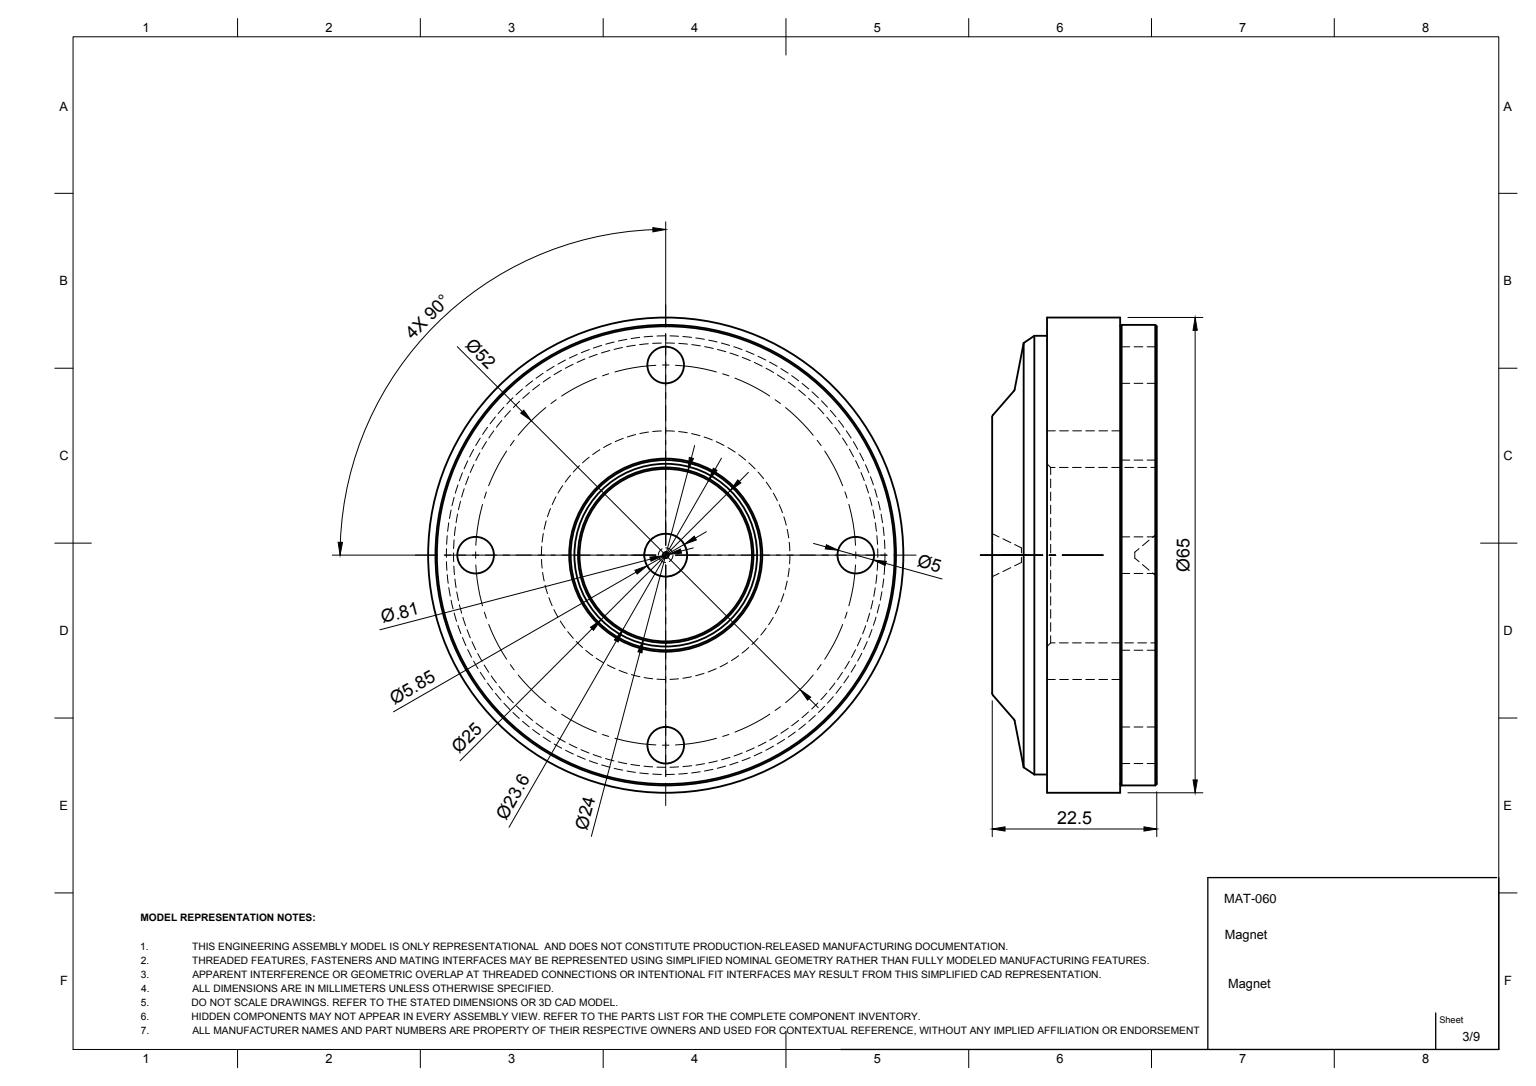
ISO-10303-21;
HEADER;
FILE_DESCRIPTION (('STEP AP214'),
    '1' );
FILE_NAME ('Magnet.step',
    '2026-10-29T23:46:56',
    ( '' ),
    ( '' ),
    'SwSTEP 2.0',
    'SolidWorks 2020',
    '' );
FILE_SCHEMA (( 'AUTOMOTIVE_DESIGN' ));
ENDSEC;

DATA;
#2=VECTOR ( 'NONE', #10897, 1000.000000000000000 ) ;
#14=CONICAL_SURFACE ( 'NONE', #3681, 2.923537884824412014, 0.6981317007977324574 ) ;
#45=AXIS2_PLACEMENT_3D ( 'NONE', #7239, #26769, #16743 ) ;
#47=VECTOR ( 'NONE', #22684, 1000.000000000000114 ) ;
#71=ORIENTED_EDGE ( 'NONE', *, *, #26696, .T. ) ;
#91=AXIS2_PLACEMENT_3D ( 'NONE', #3983, #26796, #16125 ) ;
#98=CONICAL_SURFACE ( 'NONE', #18421, 11.79999999999997762, 0.7853981633974786991 ) ;
#100=VECTOR ( 'NONE', #2675, 1000.000000000000114 ) ;
#109=FACE_OUTER_BOUND ( 'NONE', #5838, .T. ) ;
#111=DIRECTION ( 'NONE',  ( -0.000000000000000000, 1.000000000000000000, -0.000000000000000000 ) ) ;
#122=EDGE_CURVE ( 'NONE', #19617, #28878, #29198, .T. ) ;
#132=DIRECTION ( 'NONE',  ( 0.000000000000000000, 0.000000000000000000, -1.000000000000000000 ) ) ;
#244=VECTOR ( 'NONE', #7734, 1000.000000000000114 ) ;
#252=LINE ( 'NONE', #27506, #6964 ) ;
#257=VERTEX_POINT ( 'NONE', #4514 ) ;
#265=FACE_OUTER_BOUND ( 'NONE', #5953, .T. ) ;
#277=ORIENTED_EDGE ( 'NONE', *, *, #29434, .F. ) ;
#296=AXIS2_PLACEMENT_3D ( 'NONE', #20204, #23316, #10529 ) ;
#298=EDGE_CURVE ( 'NONE', #8568, #25382, #4926, .T. ) ;
#348=DIRECTION ( 'NONE',  ( -0.000000000000000000, -1.000000000000000000, -0.000000000000000000 ) ) ;
#447=ORIENTED_EDGE ( 'NONE', *, *, #29161, .T. ) ;
#459=ORIENTED_EDGE ( 'NONE', *, *, #23712, .T. ) ;
#483=ADVANCED_FACE ( 'NONE', ( #7004 ), #4048, .T. ) ;
#496=LINE ( 'NONE', #32361, #244 ) ;
#502=DIRECTION ( 'NONE',  ( 0.000000000000000000, 0.000000000000000000, 1.000000000000000000 ) ) ;
#538=ORIENTED_EDGE ( 'NONE', *, *, #31344, .T. ) ;
#605=DIRECTION ( 'NONE',  ( 0.000000000000000000, -1.000000000000000000, 0.000000000000000000 ) ) ;
#622=CIRCLE ( 'NONE', #1640, 30.00000000000000000 ) ;
#636=FACE_OUTER_BOUND ( 'NONE', #28736, .T. ) ;
#638=ORIENTED_EDGE ( 'NONE', *, *, #25897, .T. ) ;
#686=ORIENTED_EDGE ( 'NONE', *, *, #11571, .F. ) ;
#691=ORIENTED_EDGE ( 'NONE', *, *, #20114, .F. ) ;
#732=ORIENTED_EDGE ( 'NONE', *, *, #12775, .F. ) ;
#759=PLANE ( 'NONE',  #9679 ) ;
#765=CARTESIAN_POINT ( 'NONE',  ( 21.09785597605719332, 30.56454579224779522, 47.04930799450051637 ) ) ;
#768=DIRECTION ( 'NONE',  ( -0.000000000000000000, -1.000000000000000000, -0.000000000000000000 ) ) ;
#814=CYLINDRICAL_SURFACE ( 'NONE', #19867, 2.499999999999998668 ) ;
#816=EDGE_LOOP ( 'NONE', ( #11067, #9782, #2400, #22463 ) ) ;
#819=ADVANCED_FACE ( 'NONE', ( #7090 ), #4794, .F. ) ;
#883=CARTESIAN_POINT ( 'NONE',  ( 21.09785597605719332, 30.56454579224779522, 47.04930799450051637 ) ) ;
#932=ORIENTED_EDGE ( 'NONE', *, *, #25282, .F. ) ;
#939=AXIS2_PLACEMENT_3D ( 'NONE', #4537, #12591, #24892 ) ;
#952=VECTOR ( 'NONE', #28444, 1000.000000000000114 ) ;
#1011=CARTESIAN_POINT ( 'NONE',  ( 21.09785597605719687, 43.75535478762431296, 76.06768081105269630 ) ) ;
#1060=ORIENTED_EDGE ( 'NONE', *, *, #12224, .F. ) ;
#1066=STYLED_ITEM('',(#32522),#12454);
#1071=ORIENTED_EDGE ( 'NONE', *, *, #23936, .F. ) ;
#1082=CARTESIAN_POINT ( 'NONE',  ( 21.09785597605719332, 40.56454579224780588, 47.04930799450051637 ) ) ;
#1089=EDGE_LOOP ( 'NONE', ( #31480, #28380, #1599, #4895 ) ) ;
#1092=CARTESIAN_POINT ( 'NONE',  ( 21.09785597605719332, 40.06454579224778456, 47.04930799450051637 ) ) ;
#1118=EDGE_LOOP ( 'NONE', ( #1286, #26031, #11888, #26251 ) ) ;
#1132=AXIS2_PLACEMENT_3D ( 'NONE', #16655, #9285, #24220 ) ;
#1146=CIRCLE ( 'NONE', #29981, 12.50000000000001776 ) ;
#1173=VECTOR ( 'NONE', #9327, 1000.000000000000000 ) ;
#1185=ADVANCED_FACE ( 'NONE', ( #16721 ), #7215, .T. ) ;
#1203=EDGE_LOOP ( 'NONE', ( #5817, #15284, #10647, #19677 ) ) ;
#1217=VECTOR ( 'NONE', #18449, 1000.000000000000000 ) ;
#1226=CARTESIAN_POINT ( 'NONE',  ( 21.09785597605719332, 30.36454579224779238, 47.04930799450051637 ) ) ;
#1235=DIRECTION ( 'NONE',  ( 0.000000000000000000, 0.000000000000000000, 1.000000000000000000 ) ) ;
#1286=ORIENTED_EDGE ( 'NONE', *, *, #27316, .F. ) ;
#1292=EDGE_LOOP ( 'NONE', ( #17485, #2942, #9544, #30462 ) ) ;
#1300=AXIS2_PLACEMENT_3D ( 'NONE', #24449, #4434, #31842 ) ;
#1313=EDGE_LOOP ( 'NONE', ( #3808, #4252, #18593, #32168 ) ) ;
#1333=COLOUR_RGB ( '',0.7921568627450980005, 0.8196078431372548767, 0.9333333333333333481 ) ;
#1342=CARTESIAN_POINT ( 'NONE',  ( 21.09785597605719332, 30.56454579224779522, 15.74930799450053520 ) ) ;
#1354=DIRECTION ( 'NONE',  ( 0.000000000000000000, 0.000000000000000000, 1.000000000000000000 ) ) ;
#1359=EDGE_CURVE ( 'NONE', #12063, #12175, #10176, .T. ) ;
#1389=CARTESIAN_POINT ( 'NONE',  ( 21.09785597605719332, 30.56454579224779522, 33.84930799450050642 ) ) ;
#1408=DIRECTION ( 'NONE',  ( -0.000000000000000000, 1.000000000000000000, -0.000000000000000000 ) ) ;
#1416=EDGE_CURVE ( 'NONE', #25267, #14096, #7468, .T. ) ;
#1442=DIRECTION ( 'NONE',  ( 0.000000000000000000, 0.000000000000000000, 1.000000000000000000 ) ) ;
#1444=AXIS2_PLACEMENT_3D ( 'NONE', #20383, #7445, #27619 ) ;
#1449=EDGE_LOOP ( 'NONE', ( #4769, #28960 ) ) ;
#1462=DIRECTION ( 'NONE',  ( 0.000000000000000000, 0.000000000000000000, -1.000000000000000000 ) ) ;
#1504=DIRECTION ( 'NONE',  ( 0.000000000000000000, -0.000000000000000000, -1.000000000000000000 ) ) ;
#1516=FILL_AREA_STYLE ('',( #3660 ) ) ;
#1564=VERTEX_POINT ( 'NONE', #24406 ) ;
#1575=ORIENTED_EDGE ( 'NONE', *, *, #22675, .F. ) ;
#1598=AXIS2_PLACEMENT_3D ( 'NONE', #20368, #5295, #15139 ) ;
#1599=ORIENTED_EDGE ( 'NONE', *, *, #28935, .T. ) ;
#1601=PLANE ( 'NONE',  #30450 ) ;
#1625=AXIS2_PLACEMENT_3D ( 'NONE', #26803, #31574, #31889 ) ;
#1633=ORIENTED_EDGE ( 'NONE', *, *, #8614, .T. ) ;
#1640=AXIS2_PLACEMENT_3D ( 'NONE', #1082, #605, #20783 ) ;
#1645=AXIS2_PLACEMENT_3D ( 'NONE', #2215, #7303, #27489 ) ;
#1727=DIRECTION ( 'NONE',  ( 0.000000000000000000, 0.000000000000000000, 1.000000000000000000 ) ) ;
#1779=EDGE_CURVE ( 'NONE', #24681, #28894, #7495, .T. ) ;
#1787=DIRECTION ( 'NONE',  ( 0.000000000000000000, 0.000000000000000000, -1.000000000000000000 ) ) ;
#1790=VERTEX_POINT ( 'NONE', #20937 ) ;
#1801=EDGE_CURVE ( 'NONE', #17244, #15830, #19463, .T. ) ;
#1816=EDGE_CURVE ( 'NONE', #22757, #5318, #622, .T. ) ;
#1839=ADVANCED_FACE ( 'NONE', ( #31129, #10942 ), #30649, .T. ) ;
#1877=AXIS2_PLACEMENT_3D ( 'NONE', #16713, #9184, #26743 ) ;
#1887=FACE_OUTER_BOUND ( 'NONE', #17720, .T. ) ;
#1919=EDGE_LOOP ( 'NONE', ( #1575, #9249, #30657, #15820 ) ) ;
#1961=AXIS2_PLACEMENT_3D ( 'NONE', #13939, #11633, #11953 ) ;
#1975=ORIENTED_EDGE ( 'NONE', *, *, #7569, .F. ) ;
#1985=EDGE_CURVE ( 'NONE', #6454, #6391, #27880, .T. ) ;
#1987=AXIS2_PLACEMENT_3D ( 'NONE', #8912, #6617, #21212 ) ;
#2008=FACE_OUTER_BOUND ( 'NONE', #5670, .T. ) ;
#2035=EDGE_LOOP ( 'NONE', ( #28490, #17099, #19281, #32413 ) ) ;
#2068=AXIS2_PLACEMENT_3D ( 'NONE', #7531, #10318, #15399 ) ;
#2095=DIRECTION ( 'NONE',  ( 0.000000000000000000, 0.000000000000000000, -1.000000000000000000 ) ) ;
#2121=DIRECTION ( 'NONE',  ( -0.000000000000000000, -1.000000000000000000, -0.000000000000000000 ) ) ;
#2136=DIRECTION ( 'NONE',  ( 0.000000000000000000, 1.000000000000000000, 0.000000000000000000 ) ) ;
#2162=DIRECTION ( 'NONE',  ( 0.000000000000000000, 0.000000000000000000, 1.000000000000000000 ) ) ;
#2215=CARTESIAN_POINT ( 'NONE',  ( 21.09785597605719332, 30.36454579224779238, 47.04930799450051637 ) ) ;
#2245=FACE_BOUND ( 'NONE', #17285, .T. ) ;
#2286=VERTEX_POINT ( 'NONE', #12813 ) ;
#2314=PLANE ( 'NONE',  #32485 ) ;
#2325=AXIS2_PLACEMENT_3D ( 'NONE', #7259, #22180, #32208 ) ;
#2337=DIRECTION ( 'NONE',  ( 0.000000000000000000, 1.000000000000000000, 0.000000000000000000 ) ) ;
#2354=ORIENTED_EDGE ( 'NONE', *, *, #13031, .T. ) ;
#2355=EDGE_LOOP ( 'NONE', ( #9054, #15659, #16923, #25728 ) ) ;
#2360=AXIS2_PLACEMENT_3D ( 'NONE', #29508, #9641, #14246 ) ;
#2389=CARTESIAN_POINT ( 'NONE',  ( 21.09785597605719332, 25.56454579224779167, 33.84930799450050642 ) ) ;
#2400=ORIENTED_EDGE ( 'NONE', *, *, #2953, .T. ) ;
#2406=CARTESIAN_POINT ( 'NONE',  ( 21.09785597605719332, 48.06454579224779877, 50.00023834876391504 ) ) ;
#2432=EDGE_CURVE ( 'NONE', #5318, #19617, #8358, .T. ) ;
#2438=ORIENTED_EDGE ( 'NONE', *, *, #7569, .T. ) ;
#2466=EDGE_LOOP ( 'NONE', ( #32496, #15726, #538, #3563 ) ) ;
#2498=CARTESIAN_POINT ( 'NONE',  ( 21.09785597605719332, 40.06454579224778456, 59.04930799450051637 ) ) ;
#2505=ORIENTED_EDGE ( 'NONE', *, *, #17038, .T. ) ;
#2580=DIRECTION ( 'NONE',  ( 0.000000000000000000, 0.000000000000000000, -1.000000000000000000 ) ) ;
#2598=EDGE_CURVE ( 'NONE', #23536, #19811, #3820, .T. ) ;
#2626=ORIENTED_EDGE ( 'NONE', *, *, #122, .T. ) ;
#2658=FACE_OUTER_BOUND ( 'NONE', #25338, .T. ) ;
#2674=FACE_OUTER_BOUND ( 'NONE', #2355, .T. ) ;
#2675=DIRECTION ( 'NONE',  ( 9.242526717056601033E-17, -0.6560590289905074979, 0.7547095802227717920 ) ) ;
#2699=LINE ( 'NONE', #15019, #27764 ) ;
#2784=FACE_OUTER_BOUND ( 'NONE', #1292, .T. ) ;
#2814=EDGE_CURVE ( 'NONE', #4198, #16034, #19041, .T. ) ;
#2856=AXIS2_PLACEMENT_3D ( 'NONE', #24398, #17003, #21928 ) ;
#2867=ORIENTED_EDGE ( 'NONE', *, *, #8743, .T. ) ;
#2878=PRODUCT_DEFINITION_CONTEXT ( 'detailed design', #25444, 'design' ) ;
#2879=ORIENTED_EDGE ( 'NONE', *, *, #8848, .F. ) ;
#2893=FACE_BOUND ( 'NONE', #21626, .T. ) ;
#2924=EDGE_CURVE ( 'NONE', #9356, #12175, #6500, .T. ) ;
#2935=CIRCLE ( 'NONE', #15520, 13.00000000000000533 ) ;
#2942=ORIENTED_EDGE ( 'NONE', *, *, #6749, .F. ) ;
#2953=EDGE_CURVE ( 'NONE', #25453, #12063, #26847, .T. ) ;
#3023=CARTESIAN_POINT ( 'NONE',  ( 21.09785597605719687, 40.56454579224780588, 17.04930799450051637 ) ) ;
#3047=CARTESIAN_POINT ( 'NONE',  ( 21.09785597605719332, 42.30003263981368633, 47.04930799450051637 ) ) ;
#3112=CIRCLE ( 'NONE', #23030, 2.950930354263400890 ) ;
#3168=CARTESIAN_POINT ( 'NONE',  ( 21.09785597605719332, 25.56454579224779877, 47.04930799450051637 ) ) ;
#3178=CYLINDRICAL_SURFACE ( 'NONE', #10556, 2.500000000000002220 ) ;
#3199=AXIS2_PLACEMENT_3D ( 'NONE', #4469, #4630, #11701 ) ;
#3200=ADVANCED_FACE ( 'NONE', ( #4853 ), #25367, .F. ) ;
#3211=FACE_OUTER_BOUND ( 'NONE', #19132, .T. ) ;
#3215=ORIENTED_EDGE ( 'NONE', *, *, #6112, .T. ) ;
#3220=CARTESIAN_POINT ( 'NONE',  ( 21.09785597605719332, 30.56454579224779522, 73.04930799450052348 ) ) ;
#3299=PRODUCT ( 'Magnet', 'Magnet', '', ( #30204 ) ) ;
#3304=EDGE_LOOP ( 'NONE', ( #14921, #19098, #10073, #24712 ) ) ;
#3352=ORIENTED_EDGE ( 'NONE', *, *, #29648, .F. ) ;
#3370=ORIENTED_EDGE ( 'NONE', *, *, #21556, .T. ) ;
#3379=DIRECTION ( 'NONE',  ( 0.000000000000000000, -1.000000000000000000, 0.000000000000000000 ) ) ;
#3382=DIRECTION ( 'NONE',  ( -0.000000000000000000, -1.000000000000000000, -0.000000000000000000 ) ) ;
#3393=AXIS2_PLACEMENT_3D ( 'NONE', #22988, #25620, #502 ) ;
#3400=ADVANCED_FACE ( 'NONE', ( #20590 ), #13812, .T. ) ;
#3464=CARTESIAN_POINT ( 'NONE',  ( 21.09785597605719332, 25.56454579224779877, 49.97284587932492883 ) ) ;
#3500=DIRECTION ( 'NONE',  ( 0.000000000000000000, 0.000000000000000000, -1.000000000000000000 ) ) ;
#3529=ORIENTED_EDGE ( 'NONE', *, *, #7650, .F. ) ;
#3532=CARTESIAN_POINT ( 'NONE',  ( 21.09785597605719332, 25.56454579224779877, 47.04930799450051637 ) ) ;
#3563=ORIENTED_EDGE ( 'NONE', *, *, #8136, .T. ) ;
#3615=ORIENTED_EDGE ( 'NONE', *, *, #29434, .T. ) ;
#3660=FILL_AREA_STYLE_COLOUR ( '', #1333 ) ;
#3680=AXIS2_PLACEMENT_3D ( 'NONE', #5413, #15417, #25429 ) ;
#3681=AXIS2_PLACEMENT_3D ( 'NONE', #15156, #32392, #29939 ) ;
#3719=VECTOR ( 'NONE', #16013, 1000.000000000000000 ) ;
#3727=TOROIDAL_SURFACE ( 'NONE', #6353, 18.86195243859455672, 0.5000000000000000000 ) ;
#3731=CIRCLE ( 'NONE', #12060, 31.29999999999997229 ) ;
#3738=VERTEX_POINT ( 'NONE', #21023 ) ;
#3745=LINE ( 'NONE', #11304, #27933 ) ;
#3765=ORIENTED_EDGE ( 'NONE', *, *, #1816, .F. ) ;
#3768=FACE_OUTER_BOUND ( 'NONE', #18350, .T. ) ;
#3769=CARTESIAN_POINT ( 'NONE',  ( -4.902144023942810236, 30.56554579224779644, 44.54930799450042400 ) ) ;
#3808=ORIENTED_EDGE ( 'NONE', *, *, #30736, .F. ) ;
#3811=CARTESIAN_POINT ( 'NONE',  ( 21.09785597605719332, 30.36454579224777461, 15.54930799450051460 ) ) ;
#3820=CIRCLE ( 'NONE', #21121, 2.500000000000002220 ) ;
#3823=( NAMED_UNIT ( * ) PLANE_ANGLE_UNIT ( ) SI_UNIT ( $, .RADIAN. ) );
#3844=ADVANCED_FACE ( 'NONE', ( #32351 ), #2314, .T. ) ;
#3848=AXIS2_PLACEMENT_3D ( 'NONE', #29111, #24333, #22031 ) ;
#3870=DIRECTION ( 'NONE',  ( 0.000000000000000000, 1.000000000000000000, 0.000000000000000000 ) ) ;
#3872=DIRECTION ( 'NONE',  ( 8.659560562354931626E-17, 0.7071067811865474617, -0.7071067811865475727 ) ) ;
#3881=ORIENTED_EDGE ( 'NONE', *, *, #14421, .F. ) ;
#3913=CARTESIAN_POINT ( 'NONE',  ( 21.09785597605719332, 44.06454579224779877, 47.04930799450051637 ) ) ;
#3917=AXIS2_PLACEMENT_3D ( 'NONE', #15584, #10691, #25602 ) ;
#3919=CARTESIAN_POINT ( 'NONE',  ( 21.09785597605719332, 30.36454579224779238, 34.04930799450050927 ) ) ;
#3922=DIRECTION ( 'NONE',  ( -0.000000000000000000, -1.000000000000000000, -0.000000000000000000 ) ) ;
#3952=VERTEX_POINT ( 'NONE', #10829 ) ;
#3983=CARTESIAN_POINT ( 'NONE',  ( 21.09785597605719332, 44.06454579224779877, 47.04930799450051637 ) ) ;
#3987=FACE_OUTER_BOUND ( 'NONE', #11241, .T. ) ;
#3988=EDGE_CURVE ( 'NONE', #7332, #10562, #29362, .T. ) ;
#3991=DIRECTION ( 'NONE',  ( 0.000000000000000000, 0.000000000000000000, -1.000000000000000000 ) ) ;
#3998=DIRECTION ( 'NONE',  ( 1.202146588165213953E-16, -0.1908089953765421121, 0.9816271834476645308 ) ) ;
#4013=CARTESIAN_POINT ( 'NONE',  ( 47.09785597605719687, 30.56554579224779644, 49.54930799450078638 ) ) ;
#4043=ORIENTED_EDGE ( 'NONE', *, *, #23890, .F. ) ;
#4048=PLANE ( 'NONE',  #18437 ) ;
#4100=DIRECTION ( 'NONE',  ( 0.000000000000000000, 0.000000000000000000, -1.000000000000000000 ) ) ;
#4115=ORIENTED_EDGE ( 'NONE', *, *, #25644, .T. ) ;
#4149=EDGE_CURVE ( 'NONE', #19482, #30996, #10519, .T. ) ;
#4181=DIRECTION ( 'NONE',  ( 0.000000000000000000, 0.000000000000000000, 1.000000000000000000 ) ) ;
#4185=ORIENTED_EDGE ( 'NONE', *, *, #15938, .T. ) ;
#4198=VERTEX_POINT ( 'NONE', #19641 ) ;
#4211=VECTOR ( 'NONE', #12710, 1000.000000000000000 ) ;
#4219=EDGE_LOOP ( 'NONE', ( #12264, #18361, #29054, #29638 ) ) ;
#4221=ADVANCED_FACE ( 'NONE', ( #22270 ), #14159, .T. ) ;
#4222=DIRECTION ( 'NONE',  ( -0.000000000000000000, -1.000000000000000000, -0.000000000000000000 ) ) ;
#4225=DIRECTION ( 'NONE',  ( -0.000000000000000000, 1.000000000000000000, -0.000000000000000000 ) ) ;
#4251=DIRECTION ( 'NONE',  ( 0.000000000000000000, -1.000000000000000000, 0.000000000000000000 ) ) ;
#4252=ORIENTED_EDGE ( 'NONE', *, *, #2598, .F. ) ;
#4295=DIRECTION ( 'NONE',  ( 0.000000000000000000, 0.000000000000000000, 1.000000000000000000 ) ) ;
#4304=AXIS2_PLACEMENT_3D ( 'NONE', #7479, #29300, #27003 ) ;
#4310=AXIS2_PLACEMENT_3D ( 'NONE', #3532, #16931, #19222 ) ;
#4318=CARTESIAN_POINT ( 'NONE',  ( 21.09785597605719332, 40.56454579224779877, 47.04930799450051637 ) ) ;
#4336=CONICAL_SURFACE ( 'NONE', #15873, 31.29999999999997939, 0.7853981633974482790 ) ;
#4397=DIRECTION ( 'NONE',  ( 0.000000000000000000, 0.000000000000000000, 1.000000000000000000 ) ) ;
#4434=DIRECTION ( 'NONE',  ( 0.000000000000000000, 1.000000000000000000, 0.000000000000000000 ) ) ;
#4454=AXIS2_PLACEMENT_3D ( 'NONE', #22592, #111, #27854 ) ;
#4458=DIRECTION ( 'NONE',  ( 0.000000000000000000, -1.000000000000000000, 0.000000000000000000 ) ) ;
#4459=DIRECTION ( 'NONE',  ( -1.000000000000000000, 0.000000000000000000, 0.000000000000000000 ) ) ;
#4468=CARTESIAN_POINT ( 'NONE',  ( 21.09785597605719332, 47.94190058235918173, 47.04930799450051637 ) ) ;
#4469=CARTESIAN_POINT ( 'NONE',  ( 21.09785597605719332, 30.56454579224779522, 47.04930799450051637 ) ) ;
#4509=DIRECTION ( 'NONE',  ( 0.000000000000000000, 0.000000000000000000, 1.000000000000000000 ) ) ;
#4514=CARTESIAN_POINT ( 'NONE',  ( 21.09785597605719332, 25.56454579224779167, 60.24930799450052632 ) ) ;
#4523=ORIENTED_EDGE ( 'NONE', *, *, #1416, .F. ) ;
#4537=CARTESIAN_POINT ( 'NONE',  ( 21.09785597605719332, 25.56454579224779167, 47.04930799450051637 ) ) ;
#4575=EDGE_CURVE ( 'NONE', #14096, #28333, #31930, .T. ) ;
#4603=DIRECTION ( 'NONE',  ( 0.000000000000000000, -1.000000000000000000, 0.000000000000000000 ) ) ;
#4610=AXIS2_PLACEMENT_3D ( 'NONE', #31469, #23749, #11436 ) ;
#4630=DIRECTION ( 'NONE',  ( 0.000000000000000000, -1.000000000000000000, 0.000000000000000000 ) ) ;
#4650=DIRECTION ( 'NONE',  ( 0.000000000000000000, 0.000000000000000000, -1.000000000000000000 ) ) ;
#4661=AXIS2_PLACEMENT_3D ( 'NONE', #16707, #4251, #5184 ) ;
#4765=DIRECTION ( 'NONE',  ( 0.000000000000000000, 0.000000000000000000, -1.000000000000000000 ) ) ;
#4769=ORIENTED_EDGE ( 'NONE', *, *, #26658, .T. ) ;
#4778=CIRCLE ( 'NONE', #23111, 0.5000000000000004441 ) ;
#4792=CONICAL_SURFACE ( 'NONE', #91, 0.9999999999999731326, 0.4537856055185219284 ) ;
#4794=CYLINDRICAL_SURFACE ( 'NONE', #22047, 16.99999999999999289 ) ;
#4840=LINE ( 'NONE', #27973, #2 ) ;
#4848=PLANE ( 'NONE',  #4304 ) ;
#4853=FACE_OUTER_BOUND ( 'NONE', #31799, .T. ) ;
#4871=ORIENTED_EDGE ( 'NONE', *, *, #3988, .F. ) ;
#4893=CARTESIAN_POINT ( 'NONE',  ( 21.09785597605719687, 45.28940914544685370, 24.35070776595075515 ) ) ;
#4895=ORIENTED_EDGE ( 'NONE', *, *, #27999, .T. ) ;
#4914=ORIENTED_EDGE ( 'NONE', *, *, #28935, .F. ) ;
#4926=CIRCLE ( 'NONE', #20118, 31.50000000000000711 ) ;
#4931=ORIENTED_EDGE ( 'NONE', *, *, #31027, .T. ) ;
#4962=DIRECTION ( 'NONE',  ( -0.000000000000000000, -1.000000000000000000, -0.000000000000000000 ) ) ;
#5016=CARTESIAN_POINT ( 'NONE',  ( 21.09785597605719332, 25.76454579224776964, 47.04930799450051637 ) ) ;
#5060=CARTESIAN_POINT ( 'NONE',  ( 21.09785597605719332, 40.56454579224780588, 77.04930799450052348 ) ) ;
#5081=DIRECTION ( 'NONE',  ( -0.000000000000000000, 1.000000000000000000, 0.000000000000000000 ) ) ;
#5129=CYLINDRICAL_SURFACE ( 'NONE', #1598, 16.99999999999999289 ) ;
#5175=AXIS2_PLACEMENT_3D ( 'NONE', #26946, #23831, #1504 ) ;
#5178=CARTESIAN_POINT ( 'NONE',  ( 21.09785597605719332, 43.75535478762431296, 47.04930799450051637 ) ) ;
#5184=DIRECTION ( 'NONE',  ( 0.000000000000000000, 0.000000000000000000, -1.000000000000000000 ) ) ;
#5193=CARTESIAN_POINT ( 'NONE',  ( 21.09785597605719332, 25.56454579224779167, 60.24930799450052632 ) ) ;
#5195=VERTEX_POINT ( 'NONE', #21791 ) ;
#5208=VERTEX_POINT ( 'NONE', #19324 ) ;
#5209=FACE_OUTER_BOUND ( 'NONE', #14516, .T. ) ;
#5272=CIRCLE ( 'NONE', #28838, 2.500000000000002220 ) ;
#5295=DIRECTION ( 'NONE',  ( -0.000000000000000000, 1.000000000000000000, -0.000000000000000000 ) ) ;
#5318=VERTEX_POINT ( 'NONE', #5060 ) ;
#5338=DIRECTION ( 'NONE',  ( 0.000000000000000000, -1.000000000000000000, 0.000000000000000000 ) ) ;
#5413=CARTESIAN_POINT ( 'NONE',  ( 21.09785597605719332, 25.56454579224779167, 21.04930799450051282 ) ) ;
#5435=ORIENTED_EDGE ( 'NONE', *, *, #12257, .F. ) ;
#5489=VECTOR ( 'NONE', #32288, 1000.000000000000114 ) ;
#5554=VERTEX_POINT ( 'NONE', #10802 ) ;
#5606=CARTESIAN_POINT ( 'NONE',  ( 21.09785597605719332, 25.56454579224779877, 47.04930799450051637 ) ) ;
#5654=DIRECTION ( 'NONE',  ( -0.000000000000000000, -1.000000000000000000, -0.000000000000000000 ) ) ;
#5661=FACE_OUTER_BOUND ( 'NONE', #23654, .T. ) ;
#5670=EDGE_LOOP ( 'NONE', ( #9048, #26323, #27618, #15172 ) ) ;
#5672=AXIS2_PLACEMENT_3D ( 'NONE', #9629, #22745, #29655 ) ;
#5688=DIRECTION ( 'NONE',  ( 0.000000000000000000, -1.000000000000000000, 0.000000000000000000 ) ) ;
#5736=CARTESIAN_POINT ( 'NONE',  ( 21.09785597605719332, 44.99492099041257376, 47.04930799450051637 ) ) ;
#5741=CARTESIAN_POINT ( 'NONE',  ( 21.09785597605719332, 43.75535478762431296, 47.04930799450051637 ) ) ;
#5748=VECTOR ( 'NONE', #3998, 1000.000000000000000 ) ;
#5789=CARTESIAN_POINT ( 'NONE',  ( 21.09785597605719687, 30.56454579224779522, 14.54930799450051460 ) ) ;
#5811=AXIS2_PLACEMENT_3D ( 'NONE', #21100, #11116, #13265 ) ;
#5817=ORIENTED_EDGE ( 'NONE', *, *, #6229, .F. ) ;
#5838=EDGE_LOOP ( 'NONE', ( #12861, #28090, #20021, #25579 ) ) ;
#5855=AXIS2_PLACEMENT_3D ( 'NONE', #23260, #10799, #15876 ) ;
#5874=DIRECTION ( 'NONE',  ( -0.000000000000000000, -1.000000000000000000, -0.000000000000000000 ) ) ;
#5907=DIRECTION ( 'NONE',  ( 0.000000000000000000, 0.000000000000000000, -1.000000000000000000 ) ) ;
#5935=CONICAL_SURFACE ( 'NONE', #32123, 12.00000000000000355, 0.7853981633974466137 ) ;
#5953=EDGE_LOOP ( 'NONE', ( #24646, #2867, #26798, #22358 ) ) ;
#5977=DIRECTION ( 'NONE',  ( 1.000000000000000000, 0.000000000000000000, 0.000000000000000000 ) ) ;
#5997=AXIS2_PLACEMENT_3D ( 'NONE', #21521, #8734, #18731 ) ;
#6017=DIRECTION ( 'NONE',  ( 0.000000000000000000, -0.000000000000000000, 1.000000000000000000 ) ) ;
#6032=CIRCLE ( 'NONE', #3393, 2.950930354263400890 ) ;
#6034=CARTESIAN_POINT ( 'NONE',  ( 21.09785597605719332, 25.56454579224779167, 33.84930799450050642 ) ) ;
#6063=FACE_BOUND ( 'NONE', #12293, .T. ) ;
#6112=EDGE_CURVE ( 'NONE', #19482, #20710, #16307, .T. ) ;
#6113=ORIENTED_EDGE ( 'NONE', *, *, #12775, .T. ) ;
#6130=DIRECTION ( 'NONE',  ( -0.000000000000000000, -1.000000000000000000, -0.000000000000000000 ) ) ;
#6164=EDGE_LOOP ( 'NONE', ( #459, #13899 ) ) ;
#6229=EDGE_CURVE ( 'NONE', #15830, #17244, #19880, .T. ) ;
#6286=CARTESIAN_POINT ( 'NONE',  ( 0.000000000000000000, 0.000000000000000000, 0.000000000000000000 ) ) ;
#6310=ORIENTED_EDGE ( 'NONE', *, *, #29829, .T. ) ;
#6311=VECTOR ( 'NONE', #15099, 1000.000000000000227 ) ;
#6322=FACE_OUTER_BOUND ( 'NONE', #14016, .T. ) ;
#6353=AXIS2_PLACEMENT_3D ( 'NONE', #12902, #19938, #25032 ) ;
#6370=AXIS2_PLACEMENT_3D ( 'NONE', #30165, #3382, #23412 ) ;
#6379=EDGE_LOOP ( 'NONE', ( #12720, #25399, #4185, #71 ) ) ;
#6391=VERTEX_POINT ( 'NONE', #25600 ) ;
#6440=ORIENTED_EDGE ( 'NONE', *, *, #22675, .T. ) ;
#6454=VERTEX_POINT ( 'NONE', #15112 ) ;
#6483=DIRECTION ( 'NONE',  ( 0.000000000000000000, 0.000000000000000000, -1.000000000000000000 ) ) ;
#6500=CIRCLE ( 'NONE', #7562, 12.00000000000000355 ) ;
#6510=UNCERTAINTY_MEASURE_WITH_UNIT (LENGTH_MEASURE( 1.000000000000000082E-05 ), #21204, 'distance_accuracy_value', 'NONE');
#6545=CIRCLE ( 'NONE', #4454, 22.50178251985260758 ) ;
#6562=CARTESIAN_POINT ( 'NONE',  ( 21.09785597605719687, 40.56454579224779877, 30.04930799450051282 ) ) ;
#6604=PLANE ( 'NONE',  #5175 ) ;
#6617=DIRECTION ( 'NONE',  ( 0.000000000000000000, 1.000000000000000000, 0.000000000000000000 ) ) ;
#6636=EDGE_CURVE ( 'NONE', #24883, #22063, #9895, .T. ) ;
#6653=AXIS2_PLACEMENT_3D ( 'NONE', #27542, #5654, #132 ) ;
#6710=EDGE_CURVE ( 'NONE', #25964, #25453, #10441, .T. ) ;
#6732=CARTESIAN_POINT ( 'NONE',  ( 21.09785597605719332, 30.56454579224779522, 15.54930799450051460 ) ) ;
#6749=EDGE_CURVE ( 'NONE', #12175, #9356, #27718, .T. ) ;
#6812=DIRECTION ( 'NONE',  ( 1.000000000000000000, 0.000000000000000000, 2.775557561562892534E-15 ) ) ;
#6843=VECTOR ( 'NONE', #32265, 1000.000000000000000 ) ;
#6850=FACE_BOUND ( 'NONE', #14123, .T. ) ;
#6877=CARTESIAN_POINT ( 'NONE',  ( 21.09785597605719332, 25.56454579224779167, 47.04930799450051637 ) ) ;
#6899=DIRECTION ( 'NONE',  ( -0.000000000000000000, -1.000000000000000000, -0.000000000000000000 ) ) ;
#6902=CARTESIAN_POINT ( 'NONE',  ( 21.09785597605719332, 30.56454579224779522, 64.04930799450050927 ) ) ;
#6918=AXIS2_PLACEMENT_3D ( 'NONE', #883, #23534, #16137 ) ;
#6929=FACE_OUTER_BOUND ( 'NONE', #816, .T. ) ;
#6964=VECTOR ( 'NONE', #14710, 1000.000000000000114 ) ;
#6999=EDGE_CURVE ( 'NONE', #26617, #15153, #31107, .T. ) ;
#7004=FACE_OUTER_BOUND ( 'NONE', #8633, .T. ) ;
#7061=FACE_OUTER_BOUND ( 'NONE', #1089, .T. ) ;
#7090=FACE_OUTER_BOUND ( 'NONE', #30358, .T. ) ;
#7148=DIRECTION ( 'NONE',  ( 0.000000000000000000, 0.000000000000000000, -1.000000000000000000 ) ) ;
#7163=AXIS2_PLACEMENT_3D ( 'NONE', #16061, #7885, #30367 ) ;
#7191=CARTESIAN_POINT ( 'NONE',  ( 21.09785597605719332, 40.56454579224779877, 47.04930799450051637 ) ) ;
#7215=CYLINDRICAL_SURFACE ( 'NONE', #26964, 30.00000000000000711 ) ;
#7216=CIRCLE ( 'NONE', #12478, 29.01837281655233269 ) ;
#7227=VERTEX_POINT ( 'NONE', #9524 ) ;
#7239=CARTESIAN_POINT ( 'NONE',  ( 21.09785597605719332, 42.30003263981368633, 47.04930799450051637 ) ) ;
#7259=CARTESIAN_POINT ( 'NONE',  ( 21.09785597605719332, 40.56454579224780588, 47.04930799450051637 ) ) ;
#7291=FACE_OUTER_BOUND ( 'NONE', #21147, .T. ) ;
#7303=DIRECTION ( 'NONE',  ( 0.000000000000000000, 1.000000000000000000, 0.000000000000000000 ) ) ;
#7332=VERTEX_POINT ( 'NONE', #32006 ) ;
#7368=ORIENTED_EDGE ( 'NONE', *, *, #4575, .T. ) ;
#7389=EDGE_LOOP ( 'NONE', ( #18603, #32324, #24673, #17552 ) ) ;
#7412=CIRCLE ( 'NONE', #1625, 2.500000000000002220 ) ;
#7445=DIRECTION ( 'NONE',  ( -0.000000000000000000, -1.000000000000000000, -0.000000000000000000 ) ) ;
#7468=CIRCLE ( 'NONE', #11146, 13.00000000000000533 ) ;
#7479=CARTESIAN_POINT ( 'NONE',  ( 21.09785597605719332, 44.06454579224779877, 47.04930799450051637 ) ) ;
#7494=EDGE_CURVE ( 'NONE', #6454, #19454, #27435, .T. ) ;
#7495=CIRCLE ( 'NONE', #31526, 16.99999999999999289 ) ;
#7531=CARTESIAN_POINT ( 'NONE',  ( 21.09785597605719332, 30.56554579224779644, 73.04930799450052348 ) ) ;
#7534=CONICAL_SURFACE ( 'NONE', #4310, 11.79999999999997762, 0.7853981633974786991 ) ;
#7562=AXIS2_PLACEMENT_3D ( 'NONE', #1092, #5874, #28516 ) ;
#7569=EDGE_CURVE ( 'NONE', #10653, #22393, #21310, .T. ) ;
#7577=CARTESIAN_POINT ( 'NONE',  ( 21.09785597605719332, 40.56454579224779877, 47.04930799450051637 ) ) ;
#7631=ORIENTED_EDGE ( 'NONE', *, *, #10771, .F. ) ;
#7650=EDGE_CURVE ( 'NONE', #30366, #2286, #24947, .T. ) ;
#7652=CARTESIAN_POINT ( 'NONE',  ( 21.09785597605719332, 44.99492099041257376, 24.40795046456371153 ) ) ;
#7668=EDGE_CURVE ( 'NONE', #25453, #25964, #25988, .T. ) ;
#7669=CYLINDRICAL_SURFACE ( 'NONE', #25739, 13.00000000000000533 ) ;
#7720=ADVANCED_FACE ( 'NONE', ( #26088, #3768 ), #11479, .F. ) ;
#7734=DIRECTION ( 'NONE',  ( 8.659560562354932858E-17, -0.7071067811865474617, 0.7071067811865474617 ) ) ;
#7744=FACE_BOUND ( 'NONE', #1449, .T. ) ;
#7753=VERTEX_POINT ( 'NONE', #6562 ) ;
#7801=DIRECTION ( 'NONE',  ( 0.000000000000000000, 1.000000000000000000, 0.000000000000000000 ) ) ;
#7808=ORIENTED_EDGE ( 'NONE', *, *, #28579, .F. ) ;
#7826=CARTESIAN_POINT ( 'NONE',  ( 21.09785597605719332, 25.56454579224779877, 47.04930799450051637 ) ) ;
#7885=DIRECTION ( 'NONE',  ( 0.000000000000000000, 1.000000000000000000, 0.000000000000000000 ) ) ;
#7999=FACE_OUTER_BOUND ( 'NONE', #15040, .T. ) ;
#8056=AXIS2_PLACEMENT_3D ( 'NONE', #20654, #10975, #20969 ) ;
#8108=PRODUCT_DEFINITION ( 'UNKNOWN', '', #16576, #2878 ) ;
#8117=ORIENTED_EDGE ( 'NONE', *, *, #7494, .T. ) ;
#8122=CARTESIAN_POINT ( 'NONE',  ( 21.09785597605719687, 40.56454579224779877, 14.54930799450051460 ) ) ;
#8136=EDGE_CURVE ( 'NONE', #2286, #30366, #2935, .T. ) ;
#8142=ORIENTED_EDGE ( 'NONE', *, *, #2432, .F. ) ;
#8145=CIRCLE ( 'NONE', #12338, 2.499999999999999112 ) ;
#8153=DIRECTION ( 'NONE',  ( 0.000000000000000000, -1.000000000000000000, 0.000000000000000000 ) ) ;
#8155=DIRECTION ( 'NONE',  ( 0.000000000000000000, 0.000000000000000000, 1.000000000000000000 ) ) ;
#8160=DIRECTION ( 'NONE',  ( 0.000000000000000000, 1.000000000000000000, 0.000000000000000000 ) ) ;
#8172=AXIS2_PLACEMENT_3D ( 'NONE', #6286, #1354, #5977 ) ;
#8289=VERTEX_POINT ( 'NONE', #18574 ) ;
#8295=CIRCLE ( 'NONE', #4610, 16.99999999999999289 ) ;
#8314=CARTESIAN_POINT ( 'NONE',  ( 21.09785597605719332, 30.56454579224779522, 47.04930799450051637 ) ) ;
#8330=ORIENTED_EDGE ( 'NONE', *, *, #17614, .T. ) ;
#8358=LINE ( 'NONE', #13935, #28998 ) ;
#8359=ORIENTED_EDGE ( 'NONE', *, *, #23039, .T. ) ;
#8396=ORIENTED_EDGE ( 'NONE', *, *, #21513, .F. ) ;
#8419=EDGE_LOOP ( 'NONE', ( #1071, #20201, #2505, #13175 ) ) ;
#8421=CARTESIAN_POINT ( 'NONE',  ( 21.09785597605719332, 25.56454579224779877, 35.24930799450054053 ) ) ;
#8436=ORIENTED_EDGE ( 'NONE', *, *, #23389, .F. ) ;
#8455=AXIS2_PLACEMENT_3D ( 'NONE', #5736, #23613, #26398 ) ;
#8474=CARTESIAN_POINT ( 'NONE',  ( 21.09785597605719332, 25.76454579224776964, 78.54930799450052348 ) ) ;
#8488=CARTESIAN_POINT ( 'NONE',  ( 21.09785597605719332, 48.06454579224779877, 47.04930799450051637 ) ) ;
#8507=AXIS2_PLACEMENT_3D ( 'NONE', #4468, #14491, #32046 ) ;
#8535=EDGE_CURVE ( 'NONE', #8289, #3738, #15420, .T. ) ;
#8537=EDGE_CURVE ( 'NONE', #3738, #8289, #22773, .T. ) ;
#8543=CARTESIAN_POINT ( 'NONE',  ( 21.09785597605719332, 40.56454579224779877, 47.04930799450051637 ) ) ;
#8558=ORIENTED_EDGE ( 'NONE', *, *, #26902, .T. ) ;
#8568=VERTEX_POINT ( 'NONE', #3811 ) ;
#8600=FACE_OUTER_BOUND ( 'NONE', #1313, .T. ) ;
#8609=CARTESIAN_POINT ( 'NONE',  ( 21.09785597605719332, 40.56454579224780588, 47.04930799450051637 ) ) ;
#8612=CARTESIAN_POINT ( 'NONE',  ( 21.09785597605719332, 44.06454579224779877, 46.04930799450054479 ) ) ;
#8614=EDGE_CURVE ( 'NONE', #28505, #5195, #14915, .T. ) ;
#8629=CIRCLE ( 'NONE', #20152, 2.500000000000002220 ) ;
#8633=EDGE_LOOP ( 'NONE', ( #25859, #14377 ) ) ;
#8641=FACE_OUTER_BOUND ( 'NONE', #2466, .T. ) ;
#8734=DIRECTION ( 'NONE',  ( -0.000000000000000000, -1.000000000000000000, -0.000000000000000000 ) ) ;
#8741=CARTESIAN_POINT ( 'NONE',  ( 21.09785597605719687, 48.06454579224779877, 28.18735555590595609 ) ) ;
#8743=EDGE_CURVE ( 'NONE', #9356, #28978, #24813, .T. ) ;
#8786=ORIENTED_EDGE ( 'NONE', *, *, #25047, .F. ) ;
#8848=EDGE_CURVE ( 'NONE', #22400, #15153, #6032, .T. ) ;
#8877=DIRECTION ( 'NONE',  ( 0.000000000000000000, 0.000000000000000000, -1.000000000000000000 ) ) ;
#8910=DIRECTION ( 'NONE',  ( 0.000000000000000000, 0.000000000000000000, -1.000000000000000000 ) ) ;
#8912=CARTESIAN_POINT ( 'NONE',  ( 21.09785597605719332, 25.76454579224781227, 47.04930799450051637 ) ) ;
#8914=DIRECTION ( 'NONE',  ( 0.000000000000000000, -1.000000000000000000, 0.000000000000000000 ) ) ;
#8919=EDGE_LOOP ( 'NONE', ( #447, #3215, #6310, #14193 ) ) ;
#8948=ORIENTED_EDGE ( 'NONE', *, *, #23615, .F. ) ;
#8958=LINE ( 'NONE', #18952, #10526 ) ;
#8972=AXIS2_PLACEMENT_3D ( 'NONE', #17588, #4962, #10057 ) ;
#8976=CONICAL_SURFACE ( 'NONE', #5855, 30.00000000000000000, 1.378810109075523149 ) ;
#9017=AXIS2_PLACEMENT_3D ( 'NONE', #5016, #15025, #24533 ) ;
#9024=CARTESIAN_POINT ( 'NONE',  ( 21.09785597605719332, 30.56454579224779522, 47.04930799450051637 ) ) ;
#9032=CARTESIAN_POINT ( 'NONE',  ( -4.902144023942810236, 30.56554579224779644, 47.04930799450042400 ) ) ;
#9048=ORIENTED_EDGE ( 'NONE', *, *, #23668, .T. ) ;
#9054=ORIENTED_EDGE ( 'NONE', *, *, #7494, .F. ) ;
#9055=CARTESIAN_POINT ( 'NONE',  ( 21.09785597605719332, 30.36454579224777461, 47.04930799450051637 ) ) ;
#9063=CARTESIAN_POINT ( 'NONE',  ( 21.09785597605719332, 48.06454579224779877, 44.09837764023711770 ) ) ;
#9132=UNCERTAINTY_MEASURE_WITH_UNIT (LENGTH_MEASURE( 1.000000000000000082E-05 ), #26678, 'distance_accuracy_value', 'NONE');
#9184=DIRECTION ( 'NONE',  ( 0.000000000000000000, 1.000000000000000000, 0.000000000000000000 ) ) ;
#9191=DIRECTION ( 'NONE',  ( 0.000000000000000000, 0.000000000000000000, 1.000000000000000000 ) ) ;
#9205=CARTESIAN_POINT ( 'NONE',  ( 21.09785597605719332, 30.36454579224777461, 47.04930799450051637 ) ) ;
#9249=ORIENTED_EDGE ( 'NONE', *, *, #19013, .F. ) ;
#9251=DIRECTION ( 'NONE',  ( 0.000000000000000000, -1.000000000000000000, 0.000000000000000000 ) ) ;
#9271=ORIENTED_EDGE ( 'NONE', *, *, #32101, .T. ) ;
#9272=CARTESIAN_POINT ( 'NONE',  ( 21.09785597605719332, 47.94190058235918173, 47.04930799450051637 ) ) ;
#9285=DIRECTION ( 'NONE',  ( -0.000000000000000000, 1.000000000000000000, -0.000000000000000000 ) ) ;
#9305=FACE_OUTER_BOUND ( 'NONE', #16809, .T. ) ;
#9314=CARTESIAN_POINT ( 'NONE',  ( 21.09785597605719332, 28.56454579224779877, 47.04930799450051637 ) ) ;
#9325=DIRECTION ( 'NONE',  ( 0.000000000000000000, 0.000000000000000000, -1.000000000000000000 ) ) ;
#9327=DIRECTION ( 'NONE',  ( 0.000000000000000000, 0.7071067811865487940, 0.7071067811865463515 ) ) ;
#9343=FACE_OUTER_BOUND ( 'NONE', #13922, .T. ) ;
#9356=VERTEX_POINT ( 'NONE', #26542 ) ;
#9413=ORIENTED_EDGE ( 'NONE', *, *, #11572, .T. ) ;
#9424=AXIS2_PLACEMENT_3D ( 'NONE', #14672, #24842, #25003 ) ;
#9445=DIRECTION ( 'NONE',  ( 0.000000000000000000, 0.000000000000000000, 1.000000000000000000 ) ) ;
#9524=CARTESIAN_POINT ( 'NONE',  ( 21.09785597605719332, 25.56454579224779167, 75.54930799450052348 ) ) ;
#9540=EDGE_LOOP ( 'NONE', ( #12770, #24701 ) ) ;
#9544=ORIENTED_EDGE ( 'NONE', *, *, #30484, .T. ) ;
#9556=DIRECTION ( 'NONE',  ( 0.000000000000000000, 0.000000000000000000, 1.000000000000000000 ) ) ;
#9557=ADVANCED_FACE ( 'NONE', ( #6850, #2245, #19794, #11931, #9305, #29326 ), #16849, .F. ) ;
#9561=CARTESIAN_POINT ( 'NONE',  ( 21.09785597605719332, 30.56454579224779522, 15.74930799450053520 ) ) ;
#9565=CARTESIAN_POINT ( 'NONE',  ( 47.09785597605719687, 30.56454579224779522, 44.54930799450078638 ) ) ;
#9574=EDGE_CURVE ( 'NONE', #2286, #1790, #22094, .T. ) ;
#9588=ORIENTED_EDGE ( 'NONE', *, *, #12951, .T. ) ;
#9628=VECTOR ( 'NONE', #20725, 1000.000000000000114 ) ;
#9629=CARTESIAN_POINT ( 'NONE',  ( 21.09785597605719332, 40.06454579224778456, 47.04930799450051637 ) ) ;
#9641=DIRECTION ( 'NONE',  ( 0.000000000000000000, -1.000000000000000000, 0.000000000000000000 ) ) ;
#9647=DIRECTION ( 'NONE',  ( 0.000000000000000000, -1.000000000000000000, 0.000000000000000000 ) ) ;
#9648=CARTESIAN_POINT ( 'NONE',  ( 21.09785597605719332, 44.99492099041257376, 47.04930799450051637 ) ) ;
#9655=ADVANCED_FACE ( 'NONE', ( #2893, #3211 ), #759, .T. ) ;
#9679=AXIS2_PLACEMENT_3D ( 'NONE', #7826, #8153, #13081 ) ;
#9683=CIRCLE ( 'NONE', #32236, 2.500000000000002220 ) ;
#9703=ORIENTED_EDGE ( 'NONE', *, *, #15756, .T. ) ;
#9722=APPLICATION_CONTEXT ( 'automotive_design' ) ;
#9736=( GEOMETRIC_REPRESENTATION_CONTEXT ( 3 ) GLOBAL_UNCERTAINTY_ASSIGNED_CONTEXT ( ( #6510 ) ) GLOBAL_UNIT_ASSIGNED_CONTEXT ( ( #21204, #3823, #28770 ) ) REPRESENTATION_CONTEXT ( 'NONE', 'WORKASPACE' ) );
#9781=CARTESIAN_POINT ( 'NONE',  ( 21.09785597605719332, 45.28940914544685370, 47.04930799450051637 ) ) ;
#9782=ORIENTED_EDGE ( 'NONE', *, *, #7668, .F. ) ;
#9809=CARTESIAN_POINT ( 'NONE',  ( 21.09785597605719332, 25.76454579224781227, 47.04930799450051637 ) ) ;
#9858=CIRCLE ( 'NONE', #15604, 2.500000000000002220 ) ;
#9895=CIRCLE ( 'NONE', #17728, 32.50000000000000000 ) ;
#9907=EDGE_CURVE ( 'NONE', #25382, #11408, #10213, .T. ) ;
#9909=LINE ( 'NONE', #10241, #14850 ) ;
#9916=AXIS2_PLACEMENT_3D ( 'NONE', #9024, #22134, #9191 ) ;
#9947=DIRECTION ( 'NONE',  ( -0.000000000000000000, -1.000000000000000000, -0.000000000000000000 ) ) ;
#10042=DIRECTION ( 'NONE',  ( 7.871877887341991227E-17, -0.7660444431189775694, 0.6427876096865398070 ) ) ;
#10057=DIRECTION ( 'NONE',  ( 0.000000000000000000, 0.000000000000000000, 1.000000000000000000 ) ) ;
#10058=CARTESIAN_POINT ( 'NONE',  ( 21.09785597605719332, 25.56454579224779167, 47.04930799450051637 ) ) ;
#10070=CARTESIAN_POINT ( 'NONE',  ( 21.09785597605719332, 30.56554579224779644, 18.54930799450051282 ) ) ;
#10073=ORIENTED_EDGE ( 'NONE', *, *, #32357, .T. ) ;
#10122=CARTESIAN_POINT ( 'NONE',  ( 21.09785597605719687, 25.56454579224779167, 15.74930799450049257 ) ) ;
#10138=CARTESIAN_POINT ( 'NONE',  ( 21.09785597605719332, 25.76454579224779806, 60.04930799450051637 ) ) ;
#10158=EDGE_CURVE ( 'NONE', #5208, #26617, #14417, .T. ) ;
#10162=EDGE_LOOP ( 'NONE', ( #16315, #27576, #17215, #30624 ) ) ;
#10174=ADVANCED_FACE ( 'NONE', ( #31527 ), #18865, .F. ) ;
#10176=LINE ( 'NONE', #25266, #12724 ) ;
#10213=LINE ( 'NONE', #24977, #10746 ) ;
#10237=CIRCLE ( 'NONE', #2360, 30.00000000000000000 ) ;
#10241=CARTESIAN_POINT ( 'NONE',  ( 21.09785597605719332, 25.56454579224779167, 60.04930799450051637 ) ) ;
#10242=AXIS2_PLACEMENT_3D ( 'NONE', #19341, #2121, #29538 ) ;
#10286=ORIENTED_EDGE ( 'NONE', *, *, #29293, .F. ) ;
#10318=DIRECTION ( 'NONE',  ( -0.000000000000000000, -1.000000000000000000, -0.000000000000000000 ) ) ;
#10338=CARTESIAN_POINT ( 'NONE',  ( 21.09785597605719332, 44.06454579224779877, 48.04930799450048795 ) ) ;
#10358=FACE_OUTER_BOUND ( 'NONE', #11483, .T. ) ;
#10375=FACE_OUTER_BOUND ( 'NONE', #13611, .T. ) ;
#10429=DIRECTION ( 'NONE',  ( 0.000000000000000000, 0.000000000000000000, -1.000000000000000000 ) ) ;
#10441=CIRCLE ( 'NONE', #4661, 11.79999999999997762 ) ;
#10519=CIRCLE ( 'NONE', #24106, 22.64135752993680484 ) ;
#10526=VECTOR ( 'NONE', #14054, 1000.000000000000000 ) ;
#10529=DIRECTION ( 'NONE',  ( 0.000000000000000000, 0.000000000000000000, 1.000000000000000000 ) ) ;
#10547=AXIS2_PLACEMENT_3D ( 'NONE', #19320, #11790, #2095 ) ;
#10556=AXIS2_PLACEMENT_3D ( 'NONE', #30930, #27982, #3500 ) ;
#10562=VERTEX_POINT ( 'NONE', #11303 ) ;
#10595=AXIS2_PLACEMENT_3D ( 'NONE', #28503, #8160, #6017 ) ;
#10606=CARTESIAN_POINT ( 'NONE',  ( 21.09785597605719332, 30.56554579224779644, 23.54930799450051282 ) ) ;
#10638=AXIS2_PLACEMENT_3D ( 'NONE', #5606, #20537, #28733 ) ;
#10647=ORIENTED_EDGE ( 'NONE', *, *, #27239, .T. ) ;
#10653=VERTEX_POINT ( 'NONE', #24575 ) ;
#10691=DIRECTION ( 'NONE',  ( 0.000000000000000000, 1.000000000000000000, 0.000000000000000000 ) ) ;
#10742=DIRECTION ( 'NONE',  ( -0.000000000000000000, 1.000000000000000000, -0.000000000000000000 ) ) ;
#10746=VECTOR ( 'NONE', #348, 1000.000000000000000 ) ;
#10762=LINE ( 'NONE', #3023, #12062 ) ;
#10768=EDGE_LOOP ( 'NONE', ( #24611, #14453 ) ) ;
#10771=EDGE_CURVE ( 'NONE', #31740, #16313, #3731, .T. ) ;
#10799=DIRECTION ( 'NONE',  ( -0.000000000000000000, -1.000000000000000000, -0.000000000000000000 ) ) ;
#10802=CARTESIAN_POINT ( 'NONE',  ( 21.09785597605719332, 25.56454579224779877, 44.12577010967610391 ) ) ;
#10829=CARTESIAN_POINT ( 'NONE',  ( 21.09785597605719332, 47.94190058235918173, 27.85932604141070001 ) ) ;
#10839=CARTESIAN_POINT ( 'NONE',  ( 21.09785597605719332, 30.56554579224779644, 21.04930799450051282 ) ) ;
#10842=DIRECTION ( 'NONE',  ( 0.000000000000000000, 0.000000000000000000, 1.000000000000000000 ) ) ;
#10897=DIRECTION ( 'NONE',  ( -0.000000000000000000, -1.000000000000000000, -0.000000000000000000 ) ) ;
#10942=FACE_OUTER_BOUND ( 'NONE', #19087, .T. ) ;
#10944=CARTESIAN_POINT ( 'NONE',  ( 21.09785597605719687, 30.36454579224777461, 78.54930799450052348 ) ) ;
#10967=EDGE_CURVE ( 'NONE', #22393, #30811, #31609, .T. ) ;
#10975=DIRECTION ( 'NONE',  ( 1.000000000000000000, -0.000000000000000000, 1.224646799147353207E-16 ) ) ;
#11019=CONICAL_SURFACE ( 'NONE', #30390, 13.00000000000000533, 0.7853981633974482790 ) ;
#11066=SHAPE_REPRESENTATION_RELATIONSHIP ( 'NONE' , 'NONE' ,  #12446, #26470 ) ;
#11067=ORIENTED_EDGE ( 'NONE', *, *, #17614, .F. ) ;
#11085=AXIS2_PLACEMENT_3D ( 'NONE', #4893, #19980, #27865 ) ;
#11116=DIRECTION ( 'NONE',  ( -0.000000000000000000, -1.000000000000000000, -0.000000000000000000 ) ) ;
#11124=ORIENTED_EDGE ( 'NONE', *, *, #4575, .F. ) ;
#11144=DIRECTION ( 'NONE',  ( -0.000000000000000000, -1.000000000000000000, -0.000000000000000000 ) ) ;
#11146=AXIS2_PLACEMENT_3D ( 'NONE', #13765, #11144, #16053 ) ;
#11189=CARTESIAN_POINT ( 'NONE',  ( 21.09785597605719332, 25.56454579224779877, 47.04930799450051637 ) ) ;
#11203=FACE_OUTER_BOUND ( 'NONE', #4219, .T. ) ;
#11241=EDGE_LOOP ( 'NONE', ( #732, #6440, #13404, #8436 ) ) ;
#11265=FACE_OUTER_BOUND ( 'NONE', #17695, .T. ) ;
#11282=AXIS2_PLACEMENT_3D ( 'NONE', #765, #18473, #17995 ) ;
#11303=CARTESIAN_POINT ( 'NONE',  ( 21.09785597605719332, 25.56454579224779167, 23.54930799450051282 ) ) ;
#11304=CARTESIAN_POINT ( 'NONE',  ( 21.09785597605719332, 30.56554579224779644, 70.54930799450050927 ) ) ;
#11310=CARTESIAN_POINT ( 'NONE',  ( 21.09785597605719332, 44.06454579224779877, 46.04930799450054479 ) ) ;
#11312=AXIS2_PLACEMENT_3D ( 'NONE', #11654, #31032, #21155 ) ;
#11342=AXIS2_PLACEMENT_3D ( 'NONE', #3913, #31812, #1442 ) ;
#11359=CIRCLE ( 'NONE', #11342, 0.9999999999999731326 ) ;
#11374=DIRECTION ( 'NONE',  ( 0.000000000000000000, -1.000000000000000000, 0.000000000000000000 ) ) ;
#11395=CARTESIAN_POINT ( 'NONE',  ( 21.09785597605719332, 30.36454579224779238, 47.04930799450051637 ) ) ;
#11404=DIRECTION ( 'NONE',  ( 0.000000000000000000, -1.000000000000000000, 0.000000000000000000 ) ) ;
#11408=VERTEX_POINT ( 'NONE', #12598 ) ;
#11409=CARTESIAN_POINT ( 'NONE',  ( 47.09785597605719687, 25.56454579224779167, 47.04930799450078638 ) ) ;
#11419=ORIENTED_EDGE ( 'NONE', *, *, #18724, .F. ) ;
#11420=CARTESIAN_POINT ( 'NONE',  ( 21.09785597605719332, 45.06299627138002251, 47.04930799450051637 ) ) ;
#11423=ADVANCED_FACE ( 'NONE', ( #109 ), #7669, .F. ) ;
#11436=DIRECTION ( 'NONE',  ( 0.000000000000000000, 0.000000000000000000, 1.000000000000000000 ) ) ;
#11479=PLANE ( 'NONE',  #24421 ) ;
#11483=EDGE_LOOP ( 'NONE', ( #4523, #28764, #25892, #11124 ) ) ;
#11498=VECTOR ( 'NONE', #30791, 1000.000000000000000 ) ;
#11522=EDGE_CURVE ( 'NONE', #10653, #11408, #28497, .T. ) ;
#11556=DIRECTION ( 'NONE',  ( 5.368498217537939937E-17, 0.8987940462991685919, -0.4383711467890740732 ) ) ;
#11559=AXIS2_PLACEMENT_3D ( 'NONE', #12916, #17982, #18137 ) ;
#11571=EDGE_CURVE ( 'NONE', #12727, #5195, #4778, .T. ) ;
#11572=EDGE_CURVE ( 'NONE', #28878, #19617, #22573, .T. ) ;
#11591=DIRECTION ( 'NONE',  ( 0.000000000000000000, 0.000000000000000000, -1.000000000000000000 ) ) ;
#11608=CLOSED_SHELL ( 'NONE', ( #22470, #24065, #25471, #14041, #25856, #25389, #10174, #20191, #23709, #29913, #21667, #4221, #11423, #21920, #819, #32093, #27636, #12047, #15801, #29617, #1185, #29807, #19238, #1839, #17742, #31830, #13753, #25415, #3200, #25609, #21354, #3400, #20803, #17693, #7720, #12239, #28984, #19892, #9557, #25458, #29649, #20970, #16610, #11757, #28206, #12640, #13401, #14351, #483, #15081, #24906, #3844, #24649, #20601, #9655, #16260, #16432, #16779, #18293 ) ) ;
#11633=DIRECTION ( 'NONE',  ( -0.000000000000000000, -1.000000000000000000, -0.000000000000000000 ) ) ;
#11654=CARTESIAN_POINT ( 'NONE',  ( 21.09785597605719332, 25.56454579224779877, 47.04930799450051637 ) ) ;
#11666=LINE ( 'NONE', #6732, #23094 ) ;
#11670=ORIENTED_EDGE ( 'NONE', *, *, #9907, .T. ) ;
#11701=DIRECTION ( 'NONE',  ( 0.000000000000000000, -0.000000000000000000, -1.000000000000000000 ) ) ;
#11757=ADVANCED_FACE ( 'NONE', ( #16971 ), #15806, .F. ) ;
#11790=DIRECTION ( 'NONE',  ( 0.000000000000000000, -1.000000000000000000, 0.000000000000000000 ) ) ;
#11800=LINE ( 'NONE', #21795, #1173 ) ;
#11816=FACE_OUTER_BOUND ( 'NONE', #1919, .T. ) ;
#11831=CYLINDRICAL_SURFACE ( 'NONE', #18367, 31.50000000000000000 ) ;
#11854=DIRECTION ( 'NONE',  ( 0.000000000000000000, 0.000000000000000000, 1.000000000000000000 ) ) ;
#11857=DIRECTION ( 'NONE',  ( -0.000000000000000000, 1.000000000000000000, -0.000000000000000000 ) ) ;
#11863=PLANE ( 'NONE',  #3199 ) ;
#11870=ORIENTED_EDGE ( 'NONE', *, *, #1359, .T. ) ;
#11888=ORIENTED_EDGE ( 'NONE', *, *, #28579, .T. ) ;
#11920=AXIS2_PLACEMENT_3D ( 'NONE', #7191, #26403, #9325 ) ;
#11924=ORIENTED_EDGE ( 'NONE', *, *, #29161, .F. ) ;
#11931=FACE_BOUND ( 'NONE', #21143, .T. ) ;
#11950=FACE_OUTER_BOUND ( 'NONE', #1203, .T. ) ;
#11953=DIRECTION ( 'NONE',  ( 0.000000000000000000, 0.000000000000000000, 1.000000000000000000 ) ) ;
#11969=LINE ( 'NONE', #5193, #30430 ) ;
#11997=FACE_OUTER_BOUND ( 'NONE', #1118, .T. ) ;
#12002=VECTOR ( 'NONE', #25575, 1000.000000000000000 ) ;
#12047=ADVANCED_FACE ( 'NONE', ( #23524 ), #4792, .F. ) ;
#12060=AXIS2_PLACEMENT_3D ( 'NONE', #32463, #22763, #25551 ) ;
#12062=VECTOR ( 'NONE', #23380, 1000.000000000000000 ) ;
#12063=VERTEX_POINT ( 'NONE', #26310 ) ;
#12115=DIRECTION ( 'NONE',  ( 0.000000000000000000, 1.000000000000000000, 0.000000000000000000 ) ) ;
#12168=CIRCLE ( 'NONE', #9017, 31.50000000000000711 ) ;
#12175=VERTEX_POINT ( 'NONE', #2498 ) ;
#12195=ORIENTED_EDGE ( 'NONE', *, *, #12359, .F. ) ;
#12224=EDGE_CURVE ( 'NONE', #13560, #9356, #13007, .T. ) ;
#12239=ADVANCED_FACE ( 'NONE', ( #10375 ), #5129, .F. ) ;
#12247=VECTOR ( 'NONE', #32451, 1000.000000000000000 ) ;
#12257=EDGE_CURVE ( 'NONE', #30366, #23695, #25786, .T. ) ;
#12264=ORIENTED_EDGE ( 'NONE', *, *, #6999, .F. ) ;
#12293=EDGE_LOOP ( 'NONE', ( #12662, #29775 ) ) ;
#12319=DIRECTION ( 'NONE',  ( 0.000000000000000000, -1.000000000000000000, 0.000000000000000000 ) ) ;
#12321=SHAPE_DEFINITION_REPRESENTATION ( #26588, #12446 ) ;
#12338=AXIS2_PLACEMENT_3D ( 'NONE', #22385, #29295, #6812 ) ;
#12344=CARTESIAN_POINT ( 'NONE',  ( 21.09785597605719332, 25.76454579224779806, 34.04930799450050927 ) ) ;
#12346=DIRECTION ( 'NONE',  ( 8.659560562354919300E-17, 0.7071067811865487940, -0.7071067811865463515 ) ) ;
#12359=EDGE_CURVE ( 'NONE', #14096, #25267, #31996, .T. ) ;
#12391=DIRECTION ( 'NONE',  ( 0.000000000000000000, -1.000000000000000000, 0.000000000000000000 ) ) ;
#12426=ORIENTED_EDGE ( 'NONE', *, *, #26795, .F. ) ;
#12446=SHAPE_REPRESENTATION ( 'Magnet', ( #8172 ), #9736 ) ;
#12454=MANIFOLD_SOLID_BREP ( 'Stock-MAT-060-1', #11608 ) ;
#12460=EDGE_CURVE ( 'NONE', #20710, #19617, #8958, .T. ) ;
#12478=AXIS2_PLACEMENT_3D ( 'NONE', #5741, #13304, #5907 ) ;
#12507=CIRCLE ( 'NONE', #1987, 12.00000000000000355 ) ;
#12511=CARTESIAN_POINT ( 'NONE',  ( 21.09785597605719332, 25.56454579224779877, 49.97284587932492883 ) ) ;
#12515=DIRECTION ( 'NONE',  ( 0.000000000000000000, 1.000000000000000000, 0.000000000000000000 ) ) ;
#12526=ORIENTED_EDGE ( 'NONE', *, *, #7668, .T. ) ;
#12531=CIRCLE ( 'NONE', #22978, 31.50000000000000711 ) ;
#12556=VERTEX_POINT ( 'NONE', #32425 ) ;
#12591=DIRECTION ( 'NONE',  ( 0.000000000000000000, 1.000000000000000000, 0.000000000000000000 ) ) ;
#12598=CARTESIAN_POINT ( 'NONE',  ( 21.09785597605719687, 25.76454579224776964, 78.54930799450052348 ) ) ;
#12615=CARTESIAN_POINT ( 'NONE',  ( 47.09785597605719687, 25.56454579224779167, 47.04930799450078638 ) ) ;
#12640=ADVANCED_FACE ( 'NONE', ( #8600 ), #3178, .F. ) ;
#12656=CARTESIAN_POINT ( 'NONE',  ( -4.902144023942810236, 25.56454579224779167, 44.54930799450042400 ) ) ;
#12662=ORIENTED_EDGE ( 'NONE', *, *, #26797, .T. ) ;
#12710=DIRECTION ( 'NONE',  ( -0.000000000000000000, 1.000000000000000000, -0.000000000000000000 ) ) ;
#12720=ORIENTED_EDGE ( 'NONE', *, *, #6112, .F. ) ;
#12724=VECTOR ( 'NONE', #5081, 1000.000000000000000 ) ;
#12727=VERTEX_POINT ( 'NONE', #21370 ) ;
#12729=DIRECTION ( 'NONE',  ( 0.000000000000000000, -0.7660444431189775694, -0.6427876096865398070 ) ) ;
#12770=ORIENTED_EDGE ( 'NONE', *, *, #16380, .F. ) ;
#12775=EDGE_CURVE ( 'NONE', #12556, #32160, #7412, .T. ) ;
#12776=EDGE_CURVE ( 'NONE', #20484, #25801, #16830, .T. ) ;
#12813=CARTESIAN_POINT ( 'NONE',  ( 21.09785597605719332, 30.36454579224779238, 60.04930799450051637 ) ) ;
#12861=ORIENTED_EDGE ( 'NONE', *, *, #1416, .T. ) ;
#12889=CONICAL_SURFACE ( 'NONE', #16003, 19.04889477833696176, 0.8552113334772211140 ) ;
#12902=CARTESIAN_POINT ( 'NONE',  ( 21.09785597605719332, 47.56454579224779877, 47.04930799450051637 ) ) ;
#12916=CARTESIAN_POINT ( 'NONE',  ( 21.09785597605719332, 30.56454579224779522, 47.04930799450051637 ) ) ;
#12951=EDGE_CURVE ( 'NONE', #20780, #28878, #17762, .T. ) ;
#12989=CARTESIAN_POINT ( 'NONE',  ( 21.09785597605719332, 25.56454579224779167, 47.04930799450051637 ) ) ;
#13007=LINE ( 'NONE', #15781, #27810 ) ;
#13031=EDGE_CURVE ( 'NONE', #19454, #5554, #32445, .T. ) ;
#13065=LINE ( 'NONE', #10606, #1217 ) ;
#13081=DIRECTION ( 'NONE',  ( 0.000000000000000000, -0.000000000000000000, -1.000000000000000000 ) ) ;
#13084=DIRECTION ( 'NONE',  ( -0.000000000000000000, -1.000000000000000000, -0.000000000000000000 ) ) ;
#13089=DIRECTION ( 'NONE',  ( 0.000000000000000000, 0.000000000000000000, 1.000000000000000000 ) ) ;
#13090=VECTOR ( 'NONE', #4222, 1000.000000000000000 ) ;
#13175=ORIENTED_EDGE ( 'NONE', *, *, #14839, .T. ) ;
#13225=CARTESIAN_POINT ( 'NONE',  ( 21.09785597605719332, 40.56454579224780588, 47.04930799450051637 ) ) ;
#13265=DIRECTION ( 'NONE',  ( 0.000000000000000000, 0.000000000000000000, 1.000000000000000000 ) ) ;
#13266=FACE_OUTER_BOUND ( 'NONE', #8919, .T. ) ;
#13304=DIRECTION ( 'NONE',  ( 0.000000000000000000, 1.000000000000000000, 0.000000000000000000 ) ) ;
#13305=FACE_OUTER_BOUND ( 'NONE', #28707, .T. ) ;
#13401=ADVANCED_FACE ( 'NONE', ( #13305 ), #814, .F. ) ;
#13404=ORIENTED_EDGE ( 'NONE', *, *, #18724, .T. ) ;
#13507=AXIS2_PLACEMENT_3D ( 'NONE', #21988, #21334, #26440 ) ;
#13531=FACE_OUTER_BOUND ( 'NONE', #22045, .T. ) ;
#13551=ORIENTED_EDGE ( 'NONE', *, *, #12257, .T. ) ;
#13555=CARTESIAN_POINT ( 'NONE',  ( 21.09785597605719687, 30.56454579224779522, 30.04930799450051282 ) ) ;
#13560=VERTEX_POINT ( 'NONE', #31816 ) ;
#13574=ORIENTED_EDGE ( 'NONE', *, *, #21653, .T. ) ;
#13611=EDGE_LOOP ( 'NONE', ( #8948, #18840, #26827, #22219 ) ) ;
#13628=EDGE_CURVE ( 'NONE', #15153, #22400, #3112, .T. ) ;
#13654=VECTOR ( 'NONE', #16401, 1000.000000000000000 ) ;
#13684=LINE ( 'NONE', #31080, #29898 ) ;
#13688=ORIENTED_EDGE ( 'NONE', *, *, #298, .F. ) ;
#13692=CARTESIAN_POINT ( 'NONE',  ( 21.09785597605719332, 25.56454579224779877, 35.24930799450054053 ) ) ;
#13706=CIRCLE ( 'NONE', #8455, 22.64135752993680484 ) ;
#13722=CONICAL_SURFACE ( 'NONE', #1132, 31.50000000000000711, 0.7853981633974482790 ) ;
#13751=EDGE_CURVE ( 'NONE', #22393, #10653, #28292, .T. ) ;
#13753=ADVANCED_FACE ( 'NONE', ( #5661 ), #15838, .T. ) ;
#13765=CARTESIAN_POINT ( 'NONE',  ( 21.09785597605719332, 25.76454579224779806, 47.04930799450051637 ) ) ;
#13780=ORIENTED_EDGE ( 'NONE', *, *, #2814, .F. ) ;
#13794=ORIENTED_EDGE ( 'NONE', *, *, #12951, .F. ) ;
#13812=CONICAL_SURFACE ( 'NONE', #3848, 30.00000000000000000, 0.5934119456780768687 ) ;
#13830=LINE ( 'NONE', #1342, #952 ) ;
#13834=VECTOR ( 'NONE', #16981, 1000.000000000000114 ) ;
#13855=VERTEX_POINT ( 'NONE', #28958 ) ;
#13874=DIRECTION ( 'NONE',  ( -0.000000000000000000, -1.000000000000000000, -0.000000000000000000 ) ) ;
#13886=CARTESIAN_POINT ( 'NONE',  ( 21.09785597605719332, 42.30003263981368633, 47.04930799450051637 ) ) ;
#13899=ORIENTED_EDGE ( 'NONE', *, *, #1985, .T. ) ;
#13922=EDGE_LOOP ( 'NONE', ( #20591, #11670, #4115, #4914 ) ) ;
#13926=( GEOMETRIC_REPRESENTATION_CONTEXT ( 3 ) GLOBAL_UNCERTAINTY_ASSIGNED_CONTEXT ( ( #25563 ) ) GLOBAL_UNIT_ASSIGNED_CONTEXT ( ( #30924, #18906, #14003 ) ) REPRESENTATION_CONTEXT ( 'NONE', 'WORKASPACE' ) );
#13930=AXIS2_PLACEMENT_3D ( 'NONE', #29290, #29625, #31440 ) ;
#13935=CARTESIAN_POINT ( 'NONE',  ( 21.09785597605719332, 40.56454579224780588, 77.04930799450052348 ) ) ;
#13939=CARTESIAN_POINT ( 'NONE',  ( 21.09785597605719332, 30.56454579224779522, 47.04930799450051637 ) ) ;
#13990=ORIENTED_EDGE ( 'NONE', *, *, #8537, .T. ) ;
#13991=DIRECTION ( 'NONE',  ( 0.000000000000000000, 0.000000000000000000, 1.000000000000000000 ) ) ;
#14003=( NAMED_UNIT ( * ) SI_UNIT ( $, .STERADIAN. ) SOLID_ANGLE_UNIT ( ) );
#14016=EDGE_LOOP ( 'NONE', ( #3529, #13551, #25733, #16917 ) ) ;
#14033=AXIS2_PLACEMENT_3D ( 'NONE', #31015, #21300, #30853 ) ;
#14036=CARTESIAN_POINT ( 'NONE',  ( 21.09785597605719332, 48.06454579224779877, 47.04930799450051637 ) ) ;
#14041=ADVANCED_FACE ( 'NONE', ( #22530 ), #14, .F. ) ;
#14054=DIRECTION ( 'NONE',  ( 6.848137993413698342E-17, -0.8290375725550389596, 0.5591929034707507906 ) ) ;
#14056=DIRECTION ( 'NONE',  ( 0.000000000000000000, 1.000000000000000000, 0.000000000000000000 ) ) ;
#14075=DIRECTION ( 'NONE',  ( 0.000000000000000000, -1.000000000000000000, 0.000000000000000000 ) ) ;
#14096=VERTEX_POINT ( 'NONE', #12344 ) ;
#14107=CARTESIAN_POINT ( 'NONE',  ( 21.09785597605719332, 40.06454579224778456, 47.04930799450051637 ) ) ;
#14123=EDGE_LOOP ( 'NONE', ( #13780, #11419 ) ) ;
#14134=DIRECTION ( 'NONE',  ( 0.000000000000000000, 0.000000000000000000, 1.000000000000000000 ) ) ;
#14159=CONICAL_SURFACE ( 'NONE', #23087, 31.50000000000000711, 0.7853981633974482790 ) ;
#14165=DIRECTION ( 'NONE',  ( 0.000000000000000000, 0.000000000000000000, 1.000000000000000000 ) ) ;
#14193=ORIENTED_EDGE ( 'NONE', *, *, #15938, .F. ) ;
#14194=AXIS2_PLACEMENT_3D ( 'NONE', #26920, #12319, #4765 ) ;
#14205=FACE_OUTER_BOUND ( 'NONE', #17169, .T. ) ;
#14246=DIRECTION ( 'NONE',  ( 0.000000000000000000, 0.000000000000000000, -1.000000000000000000 ) ) ;
#14319=DIRECTION ( 'NONE',  ( -0.000000000000000000, -1.000000000000000000, -0.000000000000000000 ) ) ;
#14348=ORIENTED_EDGE ( 'NONE', *, *, #12460, .T. ) ;
#14351=ADVANCED_FACE ( 'NONE', ( #11816 ), #18856, .F. ) ;
#14359=EDGE_CURVE ( 'NONE', #23536, #19744, #26260, .T. ) ;
#14360=CARTESIAN_POINT ( 'NONE',  ( 21.09785597605719332, 30.56454579224779522, 79.54930799450052348 ) ) ;
#14377=ORIENTED_EDGE ( 'NONE', *, *, #6229, .T. ) ;
#14409=EDGE_CURVE ( 'NONE', #28894, #24681, #16259, .T. ) ;
#14410=DIRECTION ( 'NONE',  ( -0.000000000000000000, 1.000000000000000000, -0.000000000000000000 ) ) ;
#14417=CIRCLE ( 'NONE', #1300, 0.9999999999999731326 ) ;
#14421=EDGE_CURVE ( 'NONE', #25267, #257, #11969, .T. ) ;
#14453=ORIENTED_EDGE ( 'NONE', *, *, #13628, .T. ) ;
#14473=STYLED_ITEM ( 'NONE', ( #28298 ), #26470 ) ;
#14491=DIRECTION ( 'NONE',  ( -0.000000000000000000, -1.000000000000000000, -0.000000000000000000 ) ) ;
#14516=EDGE_LOOP ( 'NONE', ( #23878, #17432, #9271, #17577 ) ) ;
#14566=EDGE_LOOP ( 'NONE', ( #17831, #3370 ) ) ;
#14588=ORIENTED_EDGE ( 'NONE', *, *, #10771, .T. ) ;
#14672=CARTESIAN_POINT ( 'NONE',  ( 21.09785597605719332, 30.56454579224779522, 73.04930799450052348 ) ) ;
#14710=DIRECTION ( 'NONE',  ( 0.000000000000000000, -0.6560590289905074979, -0.7547095802227717920 ) ) ;
#14751=CARTESIAN_POINT ( 'NONE',  ( 21.09785597605719332, 40.56454579224779877, 64.04930799450050927 ) ) ;
#14806=DIRECTION ( 'NONE',  ( 0.000000000000000000, 1.000000000000000000, 0.000000000000000000 ) ) ;
#14812=DIRECTION ( 'NONE',  ( 0.000000000000000000, 0.000000000000000000, 1.000000000000000000 ) ) ;
#14839=EDGE_CURVE ( 'NONE', #27529, #7227, #9858, .T. ) ;
#14850=VECTOR ( 'NONE', #19581, 1000.000000000000000 ) ;
#14860=DIRECTION ( 'NONE',  ( -0.000000000000000000, -1.000000000000000000, -0.000000000000000000 ) ) ;
#14869=DIRECTION ( 'NONE',  ( -0.000000000000000000, 1.000000000000000000, -0.000000000000000000 ) ) ;
#14870=CIRCLE ( 'NONE', #19030, 2.499999999999999112 ) ;
#14915=CIRCLE ( 'NONE', #23292, 18.86195243859455672 ) ;
#14921=ORIENTED_EDGE ( 'NONE', *, *, #21556, .F. ) ;
#14996=ORIENTED_EDGE ( 'NONE', *, *, #10967, .F. ) ;
#15019=CARTESIAN_POINT ( 'NONE',  ( 21.09785597605719332, 25.56454579224779877, 44.12577010967610391 ) ) ;
#15025=DIRECTION ( 'NONE',  ( -0.000000000000000000, 1.000000000000000000, -0.000000000000000000 ) ) ;
#15040=EDGE_LOOP ( 'NONE', ( #10286, #31423, #30832, #7808 ) ) ;
#15061=AXIS2_PLACEMENT_3D ( 'NONE', #13886, #31927, #9445 ) ;
#15077=CONICAL_SURFACE ( 'NONE', #1444, 2.923537884824412014, 0.6981317007977324574 ) ;
#15081=ADVANCED_FACE ( 'NONE', ( #28932 ), #6604, .T. ) ;
#15091=CONICAL_SURFACE ( 'NONE', #28717, 13.20000000000000995, 0.7853981633974612686 ) ;
#15099=DIRECTION ( 'NONE',  ( 0.000000000000000000, 0.8987940462991685919, 0.4383711467890740732 ) ) ;
#15112=CARTESIAN_POINT ( 'NONE',  ( 21.09785597605719332, 28.56454579224779877, 47.45554698579308450 ) ) ;
#15139=DIRECTION ( 'NONE',  ( 0.000000000000000000, 0.000000000000000000, 1.000000000000000000 ) ) ;
#15153=VERTEX_POINT ( 'NONE', #9063 ) ;
#15156=CARTESIAN_POINT ( 'NONE',  ( 21.09785597605719332, 25.56454579224779877, 47.04930799450051637 ) ) ;
#15172=ORIENTED_EDGE ( 'NONE', *, *, #31027, .F. ) ;
#15220=AXIS2_PLACEMENT_3D ( 'NONE', #19016, #28892, #1462 ) ;
#15284=ORIENTED_EDGE ( 'NONE', *, *, #23936, .T. ) ;
#15301=CARTESIAN_POINT ( 'NONE',  ( 21.09785597605719332, 30.36454579224779238, 34.04930799450050927 ) ) ;
#15378=ORIENTED_EDGE ( 'NONE', *, *, #1359, .F. ) ;
#15399=DIRECTION ( 'NONE',  ( 0.000000000000000000, 0.000000000000000000, -1.000000000000000000 ) ) ;
#15417=DIRECTION ( 'NONE',  ( 0.000000000000000000, -1.000000000000000000, 0.000000000000000000 ) ) ;
#15420=CIRCLE ( 'NONE', #5997, 2.499999999999998668 ) ;
#15460=ORIENTED_EDGE ( 'NONE', *, *, #29829, .F. ) ;
#15520=AXIS2_PLACEMENT_3D ( 'NONE', #11395, #18933, #26500 ) ;
#15524=ORIENTED_EDGE ( 'NONE', *, *, #13751, .T. ) ;
#15530=CARTESIAN_POINT ( 'NONE',  ( 21.09785597605719332, 47.56454579224779877, 65.91126043309506599 ) ) ;
#15536=DIRECTION ( 'NONE',  ( -0.000000000000000000, -1.000000000000000000, -0.000000000000000000 ) ) ;
#15584=CARTESIAN_POINT ( 'NONE',  ( 21.09785597605719332, 47.56454579224779877, 47.04930799450051637 ) ) ;
#15604=AXIS2_PLACEMENT_3D ( 'NONE', #25342, #12391, #20087 ) ;
#15616=DIRECTION ( 'NONE',  ( 0.000000000000000000, -0.8290375725550389596, -0.5591929034707507906 ) ) ;
#15659=ORIENTED_EDGE ( 'NONE', *, *, #23712, .F. ) ;
#15713=AXIS2_PLACEMENT_3D ( 'NONE', #16390, #20833, #10842 ) ;
#15726=ORIENTED_EDGE ( 'NONE', *, *, #12359, .T. ) ;
#15756=EDGE_CURVE ( 'NONE', #3952, #28505, #20600, .T. ) ;
#15781=CARTESIAN_POINT ( 'NONE',  ( 21.09785597605719332, 25.56454579224779877, 35.04930799450050927 ) ) ;
#15801=ADVANCED_FACE ( 'NONE', ( #636 ), #24793, .F. ) ;
#15806=CONICAL_SURFACE ( 'NONE', #1645, 13.00000000000000533, 0.7853981633974482790 ) ;
#15818=DIRECTION ( 'NONE',  ( -0.000000000000000000, 1.000000000000000000, 0.000000000000000000 ) ) ;
#15820=ORIENTED_EDGE ( 'NONE', *, *, #2814, .T. ) ;
#15830=VERTEX_POINT ( 'NONE', #16201 ) ;
#15838=CYLINDRICAL_SURFACE ( 'NONE', #26712, 30.00000000000000711 ) ;
#15873=AXIS2_PLACEMENT_3D ( 'NONE', #31364, #24450, #16900 ) ;
#15875=ORIENTED_EDGE ( 'NONE', *, *, #21513, .T. ) ;
#15876=DIRECTION ( 'NONE',  ( 0.000000000000000000, 0.000000000000000000, -1.000000000000000000 ) ) ;
#15885=ORIENTED_EDGE ( 'NONE', *, *, #8136, .F. ) ;
#15909=PLANE ( 'NONE',  #7163 ) ;
#15938=EDGE_CURVE ( 'NONE', #30996, #20780, #21607, .T. ) ;
#15970=VECTOR ( 'NONE', #12346, 1000.000000000000000 ) ;
#15981=DIRECTION ( 'NONE',  ( 0.000000000000000000, 0.000000000000000000, -1.000000000000000000 ) ) ;
#15991=DIRECTION ( 'NONE',  ( -0.000000000000000000, -1.000000000000000000, -0.000000000000000000 ) ) ;
#16003=AXIS2_PLACEMENT_3D ( 'NONE', #14036, #31759, #6483 ) ;
#16013=DIRECTION ( 'NONE',  ( 0.000000000000000000, 0.7071067811865474617, 0.7071067811865475727 ) ) ;
#16034=VERTEX_POINT ( 'NONE', #27183 ) ;
#16038=ORIENTED_EDGE ( 'NONE', *, *, #6710, .F. ) ;
#16053=DIRECTION ( 'NONE',  ( 0.000000000000000000, 0.000000000000000000, 1.000000000000000000 ) ) ;
#16061=CARTESIAN_POINT ( 'NONE',  ( 21.09785597605719332, 30.56454579224779522, 47.04930799450051637 ) ) ;
#16108=VECTOR ( 'NONE', #17927, 1000.000000000000000 ) ;
#16109=CIRCLE ( 'NONE', #1961, 13.20000000000000284 ) ;
#16114=DIRECTION ( 'NONE',  ( 0.000000000000000000, 0.000000000000000000, 1.000000000000000000 ) ) ;
#16125=DIRECTION ( 'NONE',  ( 0.000000000000000000, 0.000000000000000000, 1.000000000000000000 ) ) ;
#16130=CIRCLE ( 'NONE', #939, 13.20000000000000995 ) ;
#16137=DIRECTION ( 'NONE',  ( 0.000000000000000000, 0.000000000000000000, -1.000000000000000000 ) ) ;
#16142=DIRECTION ( 'NONE',  ( -0.000000000000000000, 1.000000000000000000, -0.000000000000000000 ) ) ;
#16201=CARTESIAN_POINT ( 'NONE',  ( 21.09785597605719332, 30.56454579224779522, 75.54930799450052348 ) ) ;
#16259=CIRCLE ( 'NONE', #11559, 16.99999999999999289 ) ;
#16260=ADVANCED_FACE ( 'NONE', ( #6929 ), #7534, .T. ) ;
#16298=EDGE_CURVE ( 'NONE', #12727, #3952, #22657, .T. ) ;
#16307=LINE ( 'NONE', #23538, #5748 ) ;
#16313=VERTEX_POINT ( 'NONE', #9561 ) ;
#16315=ORIENTED_EDGE ( 'NONE', *, *, #13751, .F. ) ;
#16380=EDGE_CURVE ( 'NONE', #19744, #23803, #14870, .T. ) ;
#16390=CARTESIAN_POINT ( 'NONE',  ( 21.09785597605719332, 25.76454579224776964, 47.04930799450051637 ) ) ;
#16397=ORIENTED_EDGE ( 'NONE', *, *, #4149, .F. ) ;
#16401=DIRECTION ( 'NONE',  ( -0.000000000000000000, -1.000000000000000000, -0.000000000000000000 ) ) ;
#16421=AXIS2_PLACEMENT_3D ( 'NONE', #9781, #14869, #17640 ) ;
#16432=ADVANCED_FACE ( 'NONE', ( #2658 ), #27767, .T. ) ;
#16484=LINE ( 'NONE', #4013, #24024 ) ;
#16570=CARTESIAN_POINT ( 'NONE',  ( 21.09785597605719332, 30.56454579224779522, 47.04930799450051637 ) ) ;
#16576=PRODUCT_DEFINITION_FORMATION_WITH_SPECIFIED_SOURCE ( 'ANY', '', #3299, .NOT_KNOWN. ) ;
#16610=ADVANCED_FACE ( 'NONE', ( #21325 ), #4336, .T. ) ;
#16655=CARTESIAN_POINT ( 'NONE',  ( 21.09785597605719332, 25.76454579224776964, 47.04930799450051637 ) ) ;
#16707=CARTESIAN_POINT ( 'NONE',  ( 21.09785597605719332, 25.56454579224779877, 47.04930799450051637 ) ) ;
#16713=CARTESIAN_POINT ( 'NONE',  ( 21.09785597605719332, 30.36454579224779238, 47.04930799450051637 ) ) ;
#16721=FACE_OUTER_BOUND ( 'NONE', #18555, .T. ) ;
#16743=DIRECTION ( 'NONE',  ( 0.000000000000000000, 0.000000000000000000, -1.000000000000000000 ) ) ;
#16759=ORIENTED_EDGE ( 'NONE', *, *, #8537, .F. ) ;
#16779=ADVANCED_FACE ( 'NONE', ( #2784 ), #5935, .T. ) ;
#16809=EDGE_LOOP ( 'NONE', ( #2438, #15524 ) ) ;
#16830=CIRCLE ( 'NONE', #25741, 32.50000000000000000 ) ;
#16849=PLANE ( 'NONE',  #2856 ) ;
#16854=ORIENTED_EDGE ( 'NONE', *, *, #32101, .F. ) ;
#16884=CYLINDRICAL_SURFACE ( 'NONE', #10242, 31.50000000000000000 ) ;
#16900=DIRECTION ( 'NONE',  ( 0.000000000000000000, 0.000000000000000000, -1.000000000000000000 ) ) ;
#16917=ORIENTED_EDGE ( 'NONE', *, *, #9574, .F. ) ;
#16923=ORIENTED_EDGE ( 'NONE', *, *, #23890, .T. ) ;
#16931=DIRECTION ( 'NONE',  ( 0.000000000000000000, 1.000000000000000000, 0.000000000000000000 ) ) ;
#16971=FACE_OUTER_BOUND ( 'NONE', #32284, .T. ) ;
#16981=DIRECTION ( 'NONE',  ( 0.000000000000000000, 0.7071067811865260344, 0.7071067811865690000 ) ) ;
#17003=DIRECTION ( 'NONE',  ( 0.000000000000000000, 1.000000000000000000, 0.000000000000000000 ) ) ;
#17038=EDGE_CURVE ( 'NONE', #17244, #27529, #3745, .T. ) ;
#17072=CARTESIAN_POINT ( 'NONE',  ( 21.09785597605719332, 30.56454579224779522, 47.04930799450051637 ) ) ;
#17083=ORIENTED_EDGE ( 'NONE', *, *, #1985, .F. ) ;
#17091=CARTESIAN_POINT ( 'NONE',  ( 21.09785597605719332, 30.56454579224779522, 47.04930799450051637 ) ) ;
#17099=ORIENTED_EDGE ( 'NONE', *, *, #23039, .F. ) ;
#17111=CARTESIAN_POINT ( 'NONE',  ( 21.09785597605719332, 25.56454579224779167, 73.04930799450052348 ) ) ;
#17169=EDGE_LOOP ( 'NONE', ( #23811, #26703, #4931, #24778 ) ) ;
#17215=ORIENTED_EDGE ( 'NONE', *, *, #25644, .F. ) ;
#17216=DIRECTION ( 'NONE',  ( -0.000000000000000000, 1.000000000000000000, -0.000000000000000000 ) ) ;
#17238=AXIS2_PLACEMENT_3D ( 'NONE', #14107, #9947, #1787 ) ;
#17244=VERTEX_POINT ( 'NONE', #18316 ) ;
#17285=EDGE_LOOP ( 'NONE', ( #4871, #16854 ) ) ;
#17311=FACE_OUTER_BOUND ( 'NONE', #31857, .T. ) ;
#17334=CIRCLE ( 'NONE', #10547, 32.50000000000000000 ) ;
#17353=DIRECTION ( 'NONE',  ( -1.000000000000000000, 0.000000000000000000, -1.110223024625155594E-14 ) ) ;
#17360=CARTESIAN_POINT ( 'NONE',  ( 21.09785597605719332, 48.06454579224779877, 47.04930799450051637 ) ) ;
#17405=CARTESIAN_POINT ( 'NONE',  ( 21.09785597605719687, 30.56454579224779522, 78.34930799450049221 ) ) ;
#17410=ORIENTED_EDGE ( 'NONE', *, *, #21424, .F. ) ;
#17432=ORIENTED_EDGE ( 'NONE', *, *, #31145, .T. ) ;
#17485=ORIENTED_EDGE ( 'NONE', *, *, #8743, .F. ) ;
#17515=DIRECTION ( 'NONE',  ( 0.000000000000000000, 0.000000000000000000, -1.000000000000000000 ) ) ;
#17517=DIRECTION ( 'NONE',  ( -0.000000000000000000, -1.000000000000000000, -0.000000000000000000 ) ) ;
#17552=ORIENTED_EDGE ( 'NONE', *, *, #8614, .F. ) ;
#17577=ORIENTED_EDGE ( 'NONE', *, *, #20572, .F. ) ;
#17588=CARTESIAN_POINT ( 'NONE',  ( 21.09785597605719332, 30.56454579224779522, 47.04930799450051637 ) ) ;
#17614=EDGE_CURVE ( 'NONE', #25964, #13560, #26132, .T. ) ;
#17640=DIRECTION ( 'NONE',  ( 0.000000000000000000, 0.000000000000000000, 1.000000000000000000 ) ) ;
#17662=CARTESIAN_POINT ( 'NONE',  ( 21.09785597605719332, 25.56454579224779167, 47.04930799450051637 ) ) ;
#17687=FACE_OUTER_BOUND ( 'NONE', #8419, .T. ) ;
#17693=ADVANCED_FACE ( 'NONE', ( #29463, #26828 ), #24361, .T. ) ;
#17695=EDGE_LOOP ( 'NONE', ( #16038, #8330, #932, #26025 ) ) ;
#17702=ORIENTED_EDGE ( 'NONE', *, *, #21702, .F. ) ;
#17720=EDGE_LOOP ( 'NONE', ( #30262, #21128 ) ) ;
#17728=AXIS2_PLACEMENT_3D ( 'NONE', #28395, #23306, #31505 ) ;
#17742=ADVANCED_FACE ( 'NONE', ( #14205 ), #12889, .T. ) ;
#17743=FACE_OUTER_BOUND ( 'NONE', #32397, .T. ) ;
#17762=LINE ( 'NONE', #18081, #22464 ) ;
#17788=CARTESIAN_POINT ( 'NONE',  ( -4.902144023942810236, 25.56454579224779167, 49.54930799450042400 ) ) ;
#17790=CIRCLE ( 'NONE', #15713, 31.50000000000000711 ) ;
#17813=AXIS2_PLACEMENT_3D ( 'NONE', #18448, #21067, #23703 ) ;
#17831=ORIENTED_EDGE ( 'NONE', *, *, #2598, .T. ) ;
#17869=EDGE_LOOP ( 'NONE', ( #17083, #8117, #2354, #4043 ) ) ;
#17882=CARTESIAN_POINT ( 'NONE',  ( 21.09785597605719332, 40.06454579224778456, 47.04930799450051637 ) ) ;
#17890=CIRCLE ( 'NONE', #21035, 18.86195243859455672 ) ;
#17903=DIRECTION ( 'NONE',  ( -0.000000000000000000, -1.000000000000000000, -0.000000000000000000 ) ) ;
#17914=CARTESIAN_POINT ( 'NONE',  ( -4.902144023942810236, 25.56454579224779167, 47.04930799450042400 ) ) ;
#17927=DIRECTION ( 'NONE',  ( -0.000000000000000000, -1.000000000000000000, -0.000000000000000000 ) ) ;
#17982=DIRECTION ( 'NONE',  ( 0.000000000000000000, 1.000000000000000000, 0.000000000000000000 ) ) ;
#17995=DIRECTION ( 'NONE',  ( 0.000000000000000000, 0.000000000000000000, 1.000000000000000000 ) ) ;
#18044=AXIS2_PLACEMENT_3D ( 'NONE', #7577, #14806, #24967 ) ;
#18081=CARTESIAN_POINT ( 'NONE',  ( 21.09785597605719332, 42.30003263981368633, 17.04930799450051637 ) ) ;
#18093=CIRCLE ( 'NONE', #29103, 2.499999999999998668 ) ;
#18110=FACE_OUTER_BOUND ( 'NONE', #27833, .T. ) ;
#18137=DIRECTION ( 'NONE',  ( 0.000000000000000000, 0.000000000000000000, 1.000000000000000000 ) ) ;
#18240=CONICAL_SURFACE ( 'NONE', #5672, 12.00000000000000355, 0.7853981633974466137 ) ;
#18274=VERTEX_POINT ( 'NONE', #22503 ) ;
#18285=ORIENTED_EDGE ( 'NONE', *, *, #11572, .F. ) ;
#18293=ADVANCED_FACE ( 'NONE', ( #7744, #17743 ), #29744, .T. ) ;
#18316=CARTESIAN_POINT ( 'NONE',  ( 21.09785597605719332, 30.56454579224779522, 70.54930799450050927 ) ) ;
#18331=ORIENTED_EDGE ( 'NONE', *, *, #19013, .T. ) ;
#18332=AXIS2_PLACEMENT_3D ( 'NONE', #31601, #11404, #21245 ) ;
#18350=EDGE_LOOP ( 'NONE', ( #26357, #12426 ) ) ;
#18355=DIRECTION ( 'NONE',  ( -0.000000000000000000, 1.000000000000000000, -0.000000000000000000 ) ) ;
#18361=ORIENTED_EDGE ( 'NONE', *, *, #10158, .F. ) ;
#18367=AXIS2_PLACEMENT_3D ( 'NONE', #16570, #26590, #4100 ) ;
#18421=AXIS2_PLACEMENT_3D ( 'NONE', #24214, #3870, #1235 ) ;
#18437=AXIS2_PLACEMENT_3D ( 'NONE', #26698, #14075, #24070 ) ;
#18448=CARTESIAN_POINT ( 'NONE',  ( 21.09785597605719332, 25.56454579224779167, 47.04930799450051637 ) ) ;
#18449=DIRECTION ( 'NONE',  ( -0.000000000000000000, -1.000000000000000000, -0.000000000000000000 ) ) ;
#18473=DIRECTION ( 'NONE',  ( -0.000000000000000000, 1.000000000000000000, -0.000000000000000000 ) ) ;
#18474=DIRECTION ( 'NONE',  ( 0.000000000000000000, 0.000000000000000000, 1.000000000000000000 ) ) ;
#18521=DIRECTION ( 'NONE',  ( 0.000000000000000000, 0.000000000000000000, -1.000000000000000000 ) ) ;
#18533=DIRECTION ( 'NONE',  ( 0.000000000000000000, -1.000000000000000000, 0.000000000000000000 ) ) ;
#18548=ORIENTED_EDGE ( 'NONE', *, *, #29059, .F. ) ;
#18554=EDGE_CURVE ( 'NONE', #5318, #22757, #10237, .T. ) ;
#18555=EDGE_LOOP ( 'NONE', ( #3765, #8558, #9413, #8142 ) ) ;
#18574=CARTESIAN_POINT ( 'NONE',  ( 21.09785597605719332, 30.56454579224779522, 23.54930799450051282 ) ) ;
#18593=ORIENTED_EDGE ( 'NONE', *, *, #14359, .T. ) ;
#18603=ORIENTED_EDGE ( 'NONE', *, *, #15756, .F. ) ;
#18651=EDGE_CURVE ( 'NONE', #13855, #18274, #6545, .T. ) ;
#18664=EDGE_LOOP ( 'NONE', ( #27685, #28175 ) ) ;
#18686=EDGE_LOOP ( 'NONE', ( #32261, #25328 ) ) ;
#18724=EDGE_CURVE ( 'NONE', #16034, #4198, #9683, .T. ) ;
#18731=DIRECTION ( 'NONE',  ( 0.000000000000000000, 0.000000000000000000, 1.000000000000000000 ) ) ;
#18840=ORIENTED_EDGE ( 'NONE', *, *, #14409, .F. ) ;
#18855=DIRECTION ( 'NONE',  ( 0.000000000000000000, -0.000000000000000000, -1.000000000000000000 ) ) ;
#18856=CYLINDRICAL_SURFACE ( 'NONE', #15220, 2.500000000000002220 ) ;
#18865=CYLINDRICAL_SURFACE ( 'NONE', #21158, 2.500000000000002220 ) ;
#18896=CIRCLE ( 'NONE', #11085, 0.3000000000000016542 ) ;
#18906=( NAMED_UNIT ( * ) PLANE_ANGLE_UNIT ( ) SI_UNIT ( $, .RADIAN. ) );
#18932=CIRCLE ( 'NONE', #21561, 12.00000000000000355 ) ;
#18933=DIRECTION ( 'NONE',  ( 0.000000000000000000, 1.000000000000000000, 0.000000000000000000 ) ) ;
#18952=CARTESIAN_POINT ( 'NONE',  ( 21.09785597605719687, 42.30003263981368633, 77.04930799450052348 ) ) ;
#18971=CARTESIAN_POINT ( 'NONE',  ( 21.09785597605719332, 25.56454579224779167, 34.04930799450050927 ) ) ;
#19013=EDGE_CURVE ( 'NONE', #32160, #12556, #19126, .T. ) ;
#19016=CARTESIAN_POINT ( 'NONE',  ( 47.09785597605719687, 30.56554579224779644, 47.04930799450078638 ) ) ;
#19030=AXIS2_PLACEMENT_3D ( 'NONE', #17914, #29746, #27930 ) ;
#19041=CIRCLE ( 'NONE', #26383, 2.500000000000002220 ) ;
#19070=CARTESIAN_POINT ( 'NONE',  ( 47.09785597605719687, 30.56554579224779644, 47.04930799450078638 ) ) ;
#19087=EDGE_LOOP ( 'NONE', ( #21444, #1633 ) ) ;
#19098=ORIENTED_EDGE ( 'NONE', *, *, #30736, .T. ) ;
#19126=CIRCLE ( 'NONE', #19652, 2.500000000000002220 ) ;
#19132=EDGE_LOOP ( 'NONE', ( #12526, #23584 ) ) ;
#19140=CARTESIAN_POINT ( 'NONE',  ( 21.09785597605719332, 45.28940914544685370, 47.04930799450051637 ) ) ;
#19193=ORIENTED_EDGE ( 'NONE', *, *, #23615, .T. ) ;
#19222=DIRECTION ( 'NONE',  ( 0.000000000000000000, 0.000000000000000000, 1.000000000000000000 ) ) ;
#19238=ADVANCED_FACE ( 'NONE', ( #2008 ), #23359, .T. ) ;
#19260=VECTOR ( 'NONE', #31633, 1000.000000000000000 ) ;
#19281=ORIENTED_EDGE ( 'NONE', *, *, #21424, .T. ) ;
#19320=CARTESIAN_POINT ( 'NONE',  ( 21.09785597605719332, 30.56454579224779522, 47.04930799450051637 ) ) ;
#19324=CARTESIAN_POINT ( 'NONE',  ( 21.09785597605719332, 44.06454579224779877, 48.04930799450048795 ) ) ;
#19341=CARTESIAN_POINT ( 'NONE',  ( 21.09785597605719332, 30.56454579224779522, 47.04930799450051637 ) ) ;
#19385=CIRCLE ( 'NONE', #18332, 0.4062389912925720714 ) ;
#19387=CARTESIAN_POINT ( 'NONE',  ( 21.09785597605719332, 30.56454579224779522, 21.04930799450051282 ) ) ;
#19414=CIRCLE ( 'NONE', #19932, 13.20000000000000995 ) ;
#19454=VERTEX_POINT ( 'NONE', #3464 ) ;
#19463=CIRCLE ( 'NONE', #24181, 2.500000000000002220 ) ;
#19482=VERTEX_POINT ( 'NONE', #20544 ) ;
#19528=CARTESIAN_POINT ( 'NONE',  ( 21.09785597605719332, 42.30003263981368633, 77.04930799450052348 ) ) ;
#19540=VECTOR ( 'NONE', #31144, 1000.000000000000000 ) ;
#19543=DIRECTION ( 'NONE',  ( -0.000000000000000000, -1.000000000000000000, -0.000000000000000000 ) ) ;
#19581=DIRECTION ( 'NONE',  ( -0.000000000000000000, 1.000000000000000000, -0.000000000000000000 ) ) ;
#19597=AXIS2_PLACEMENT_3D ( 'NONE', #19387, #14319, #11854 ) ;
#19617=VERTEX_POINT ( 'NONE', #19528 ) ;
#19624=AXIS2_PLACEMENT_3D ( 'NONE', #12989, #17903, #25454 ) ;
#19640=DIRECTION ( 'NONE',  ( 0.000000000000000000, -0.000000000000000000, -1.000000000000000000 ) ) ;
#19641=CARTESIAN_POINT ( 'NONE',  ( 47.09785597605719687, 25.56454579224779167, 44.54930799450078638 ) ) ;
#19652=AXIS2_PLACEMENT_3D ( 'NONE', #22882, #14860, #27819 ) ;
#19669=AXIS2_PLACEMENT_3D ( 'NONE', #29254, #11374, #8910 ) ;
#19677=ORIENTED_EDGE ( 'NONE', *, *, #17038, .F. ) ;
#19691=DIRECTION ( 'NONE',  ( 0.000000000000000000, -1.000000000000000000, 0.000000000000000000 ) ) ;
#19744=VERTEX_POINT ( 'NONE', #12656 ) ;
#19794=FACE_BOUND ( 'NONE', #9540, .T. ) ;
#19811=VERTEX_POINT ( 'NONE', #27739 ) ;
#19867=AXIS2_PLACEMENT_3D ( 'NONE', #10839, #28555, #18521 ) ;
#19880=CIRCLE ( 'NONE', #9424, 2.500000000000002220 ) ;
#19892=ADVANCED_FACE ( 'NONE', ( #25593, #6063 ), #15909, .T. ) ;
#19932=AXIS2_PLACEMENT_3D ( 'NONE', #10058, #2337, #29920 ) ;
#19938=DIRECTION ( 'NONE',  ( 0.000000000000000000, 1.000000000000000000, 0.000000000000000000 ) ) ;
#19980=DIRECTION ( 'NONE',  ( 1.000000000000000000, 0.000000000000000000, 1.224646799147353207E-16 ) ) ;
#20009=ORIENTED_EDGE ( 'NONE', *, *, #22300, .T. ) ;
#20021=ORIENTED_EDGE ( 'NONE', *, *, #7650, .T. ) ;
#20044=CARTESIAN_POINT ( 'NONE',  ( 21.09785597605719332, 48.06454579224779877, 47.04930799450051637 ) ) ;
#20087=DIRECTION ( 'NONE',  ( 0.000000000000000000, 0.000000000000000000, -1.000000000000000000 ) ) ;
#20114=EDGE_CURVE ( 'NONE', #26617, #5208, #11359, .T. ) ;
#20118=AXIS2_PLACEMENT_3D ( 'NONE', #9055, #4458, #13991 ) ;
#20128=ORIENTED_EDGE ( 'NONE', *, *, #26902, .F. ) ;
#20152=AXIS2_PLACEMENT_3D ( 'NONE', #26778, #19543, #2162 ) ;
#20191=ADVANCED_FACE ( 'NONE', ( #11950 ), #24920, .F. ) ;
#20201=ORIENTED_EDGE ( 'NONE', *, *, #1801, .F. ) ;
#20204=CARTESIAN_POINT ( 'NONE',  ( 21.09785597605719332, 25.56454579224779167, 47.04930799450051637 ) ) ;
#20238=EDGE_LOOP ( 'NONE', ( #8359, #14588 ) ) ;
#20368=CARTESIAN_POINT ( 'NONE',  ( 21.09785597605719332, 30.56454579224779522, 47.04930799450051637 ) ) ;
#20383=CARTESIAN_POINT ( 'NONE',  ( 21.09785597605719332, 25.56454579224779877, 47.04930799450051637 ) ) ;
#20473=( GEOMETRIC_REPRESENTATION_CONTEXT ( 3 ) GLOBAL_UNCERTAINTY_ASSIGNED_CONTEXT ( ( #9132 ) ) GLOBAL_UNIT_ASSIGNED_CONTEXT ( ( #26678, #31612, #24374 ) ) REPRESENTATION_CONTEXT ( 'NONE', 'WORKASPACE' ) );
#20484=VERTEX_POINT ( 'NONE', #26637 ) ;
#20510=AXIS2_PLACEMENT_3D ( 'NONE', #5178, #7801, #7148 ) ;
#20537=DIRECTION ( 'NONE',  ( -0.000000000000000000, 1.000000000000000000, 0.000000000000000000 ) ) ;
#20544=CARTESIAN_POINT ( 'NONE',  ( 21.09785597605719687, 44.99492099041257376, 69.69066552443730700 ) ) ;
#20559=ORIENTED_EDGE ( 'NONE', *, *, #122, .F. ) ;
#20572=EDGE_CURVE ( 'NONE', #3738, #7332, #30413, .T. ) ;
#20590=FACE_OUTER_BOUND ( 'NONE', #26820, .T. ) ;
#20591=ORIENTED_EDGE ( 'NONE', *, *, #298, .T. ) ;
#20594=DIRECTION ( 'NONE',  ( 0.000000000000000000, 0.000000000000000000, 1.000000000000000000 ) ) ;
#20600=CIRCLE ( 'NONE', #8056, 0.5000000000000004441 ) ;
#20601=ADVANCED_FACE ( 'NONE', ( #2674 ), #15077, .F. ) ;
#20618=DIRECTION ( 'NONE',  ( -1.000000000000000000, 0.000000000000000000, 0.000000000000000000 ) ) ;
#20654=CARTESIAN_POINT ( 'NONE',  ( 21.09785597605719687, 47.56454579224779877, 28.18735555590595609 ) ) ;
#20710=VERTEX_POINT ( 'NONE', #1011 ) ;
#20725=DIRECTION ( 'NONE',  ( 8.659560562355194168E-17, 0.7071067811865260344, -0.7071067811865690000 ) ) ;
#20780=VERTEX_POINT ( 'NONE', #23498 ) ;
#20783=DIRECTION ( 'NONE',  ( 0.000000000000000000, 0.000000000000000000, -1.000000000000000000 ) ) ;
#20785=DIRECTION ( 'NONE',  ( 0.000000000000000000, 0.000000000000000000, -1.000000000000000000 ) ) ;
#20803=ADVANCED_FACE ( 'NONE', ( #11997 ), #29065, .T. ) ;
#20833=DIRECTION ( 'NONE',  ( -0.000000000000000000, 1.000000000000000000, -0.000000000000000000 ) ) ;
#20911=DIRECTION ( 'NONE',  ( 0.000000000000000000, 0.000000000000000000, 1.000000000000000000 ) ) ;
#20937=CARTESIAN_POINT ( 'NONE',  ( 21.09785597605719332, 30.56454579224779522, 60.24930799450052632 ) ) ;
#20969=DIRECTION ( 'NONE',  ( 0.000000000000000000, 0.000000000000000000, -1.000000000000000000 ) ) ;
#20970=ADVANCED_FACE ( 'NONE', ( #31665 ), #15091, .F. ) ;
#21023=CARTESIAN_POINT ( 'NONE',  ( 21.09785597605719332, 30.56454579224779522, 18.54930799450051282 ) ) ;
#21035=AXIS2_PLACEMENT_3D ( 'NONE', #8488, #14056, #28990 ) ;
#21067=DIRECTION ( 'NONE',  ( -0.000000000000000000, -1.000000000000000000, -0.000000000000000000 ) ) ;
#21085=ORIENTED_EDGE ( 'NONE', *, *, #9574, .T. ) ;
#21100=CARTESIAN_POINT ( 'NONE',  ( 21.09785597605719332, 25.76454579224779806, 47.04930799450051637 ) ) ;
#21121=AXIS2_PLACEMENT_3D ( 'NONE', #26884, #21625, #4397 ) ;
#21128=ORIENTED_EDGE ( 'NONE', *, *, #20114, .T. ) ;
#21143=EDGE_LOOP ( 'NONE', ( #23024, #26495 ) ) ;
#21147=EDGE_LOOP ( 'NONE', ( #13990, #28142 ) ) ;
#21155=DIRECTION ( 'NONE',  ( 0.000000000000000000, 0.000000000000000000, -1.000000000000000000 ) ) ;
#21158=AXIS2_PLACEMENT_3D ( 'NONE', #9032, #6899, #26272 ) ;
#21191=CARTESIAN_POINT ( 'NONE',  ( 21.09785597605719332, 44.06454579224779877, 47.04930799450051637 ) ) ;
#21204=( LENGTH_UNIT ( ) NAMED_UNIT ( * ) SI_UNIT ( .MILLI., .METRE. ) );
#21212=DIRECTION ( 'NONE',  ( 0.000000000000000000, 0.000000000000000000, -1.000000000000000000 ) ) ;
#21245=DIRECTION ( 'NONE',  ( 0.000000000000000000, 0.000000000000000000, -1.000000000000000000 ) ) ;
#21269=CARTESIAN_POINT ( 'NONE',  ( -4.902144023942810236, 30.56554579224779644, 49.54930799450042400 ) ) ;
#21294=DIRECTION ( 'NONE',  ( -0.000000000000000000, -1.000000000000000000, -0.000000000000000000 ) ) ;
#21297=ORIENTED_EDGE ( 'NONE', *, *, #12460, .F. ) ;
#21300=DIRECTION ( 'NONE',  ( -0.000000000000000000, 1.000000000000000000, -0.000000000000000000 ) ) ;
#21310=CIRCLE ( 'NONE', #296, 31.30000000000002913 ) ;
#21325=FACE_OUTER_BOUND ( 'NONE', #2035, .T. ) ;
#21334=DIRECTION ( 'NONE',  ( -0.000000000000000000, 1.000000000000000000, -0.000000000000000000 ) ) ;
#21341=CIRCLE ( 'NONE', #14033, 12.50000000000001776 ) ;
#21354=ADVANCED_FACE ( 'NONE', ( #11203 ), #27170, .F. ) ;
#21370=CARTESIAN_POINT ( 'NONE',  ( 21.09785597605719687, 47.94190058235918173, 66.23928994759033628 ) ) ;
#21418=CIRCLE ( 'NONE', #9916, 31.29999999999997229 ) ;
#21424=EDGE_CURVE ( 'NONE', #16313, #8568, #13830, .T. ) ;
#21439=LINE ( 'NONE', #26380, #13090 ) ;
#21444=ORIENTED_EDGE ( 'NONE', *, *, #29648, .T. ) ;
#21513=EDGE_CURVE ( 'NONE', #13855, #19482, #28040, .T. ) ;
#21521=CARTESIAN_POINT ( 'NONE',  ( 21.09785597605719332, 30.56454579224779522, 21.04930799450051282 ) ) ;
#21549=CIRCLE ( 'NONE', #20510, 29.01837281655233269 ) ;
#21556=EDGE_CURVE ( 'NONE', #19811, #23536, #8629, .T. ) ;
#21561=AXIS2_PLACEMENT_3D ( 'NONE', #9809, #12115, #17515 ) ;
#21584=EDGE_LOOP ( 'NONE', ( #3881, #12195, #7368, #30669 ) ) ;
#21607=LINE ( 'NONE', #31641, #12247 ) ;
#21625=DIRECTION ( 'NONE',  ( -0.000000000000000000, -1.000000000000000000, -0.000000000000000000 ) ) ;
#21626=EDGE_LOOP ( 'NONE', ( #31246, #29733 ) ) ;
#21653=EDGE_CURVE ( 'NONE', #31740, #25382, #496, .T. ) ;
#21667=ADVANCED_FACE ( 'NONE', ( #10358 ), #24873, .F. ) ;
#21702=EDGE_CURVE ( 'NONE', #30447, #7753, #32202, .T. ) ;
#21778=FACE_OUTER_BOUND ( 'NONE', #6164, .T. ) ;
#21791=CARTESIAN_POINT ( 'NONE',  ( 21.09785597605719332, 48.06454579224779877, 65.91126043309506599 ) ) ;
#21795=CARTESIAN_POINT ( 'NONE',  ( 21.09785597605719332, 40.06454579224778456, 59.04930799450051637 ) ) ;
#21920=ADVANCED_FACE ( 'NONE', ( #9343 ), #16884, .T. ) ;
#21928=DIRECTION ( 'NONE',  ( 0.000000000000000000, -0.000000000000000000, 1.000000000000000000 ) ) ;
#21960=ORIENTED_EDGE ( 'NONE', *, *, #6999, .T. ) ;
#21988=CARTESIAN_POINT ( 'NONE',  ( 21.09785597605719332, 30.56454579224779522, 47.04930799450051637 ) ) ;
#21991=FACE_OUTER_BOUND ( 'NONE', #26163, .T. ) ;
#22031=DIRECTION ( 'NONE',  ( 0.000000000000000000, 0.000000000000000000, -1.000000000000000000 ) ) ;
#22045=EDGE_LOOP ( 'NONE', ( #7631, #13574, #13688, #17410 ) ) ;
#22047=AXIS2_PLACEMENT_3D ( 'NONE', #17091, #11857, #14812 ) ;
#22063=VERTEX_POINT ( 'NONE', #30345 ) ;
#22094=LINE ( 'NONE', #29661, #5489 ) ;
#22134=DIRECTION ( 'NONE',  ( 0.000000000000000000, 1.000000000000000000, 0.000000000000000000 ) ) ;
#22145=DIRECTION ( 'NONE',  ( 0.000000000000000000, 0.000000000000000000, 1.000000000000000000 ) ) ;
#22180=DIRECTION ( 'NONE',  ( 0.000000000000000000, -1.000000000000000000, 0.000000000000000000 ) ) ;
#22219=ORIENTED_EDGE ( 'NONE', *, *, #21702, .T. ) ;
#22252=EDGE_CURVE ( 'NONE', #14096, #30366, #29494, .T. ) ;
#22270=FACE_OUTER_BOUND ( 'NONE', #10162, .T. ) ;
#22300=EDGE_CURVE ( 'NONE', #7753, #30447, #8295, .T. ) ;
#22331=FACE_OUTER_BOUND ( 'NONE', #7389, .T. ) ;
#22358=ORIENTED_EDGE ( 'NONE', *, *, #30484, .F. ) ;
#22385=CARTESIAN_POINT ( 'NONE',  ( -4.902144023942810236, 25.56454579224779167, 47.04930799450042400 ) ) ;
#22393=VERTEX_POINT ( 'NONE', #10122 ) ;
#22400=VERTEX_POINT ( 'NONE', #2406 ) ;
#22430=DIRECTION ( 'NONE',  ( 0.000000000000000000, -1.000000000000000000, 0.000000000000000000 ) ) ;
#22438=EDGE_CURVE ( 'NONE', #257, #28333, #16130, .T. ) ;
#22463=ORIENTED_EDGE ( 'NONE', *, *, #25897, .F. ) ;
#22464=VECTOR ( 'NONE', #15616, 1000.000000000000000 ) ;
#22470=ADVANCED_FACE ( 'NONE', ( #265 ), #18240, .T. ) ;
#22503=CARTESIAN_POINT ( 'NONE',  ( 21.09785597605719332, 45.06299627138002251, 24.54752547464790524 ) ) ;
#22530=FACE_OUTER_BOUND ( 'NONE', #17869, .T. ) ;
#22573=CIRCLE ( 'NONE', #25209, 30.00000000000000711 ) ;
#22592=CARTESIAN_POINT ( 'NONE',  ( 21.09785597605719332, 45.06299627138002251, 47.04930799450051637 ) ) ;
#22657=CIRCLE ( 'NONE', #8507, 19.18998195308981636 ) ;
#22675=EDGE_CURVE ( 'NONE', #12556, #16034, #16484, .T. ) ;
#22684=DIRECTION ( 'NONE',  ( 8.659560562354932858E-17, 0.7071067811865474617, -0.7071067811865474617 ) ) ;
#22745=DIRECTION ( 'NONE',  ( 0.000000000000000000, 1.000000000000000000, 0.000000000000000000 ) ) ;
#22757=VERTEX_POINT ( 'NONE', #24517 ) ;
#22763=DIRECTION ( 'NONE',  ( 0.000000000000000000, 1.000000000000000000, 0.000000000000000000 ) ) ;
#22773=CIRCLE ( 'NONE', #19597, 2.499999999999998668 ) ;
#22882=CARTESIAN_POINT ( 'NONE',  ( 47.09785597605719687, 30.56454579224779522, 47.04930799450078638 ) ) ;
#22888=DIRECTION ( 'NONE',  ( -0.000000000000000000, 1.000000000000000000, -0.000000000000000000 ) ) ;
#22956=LINE ( 'NONE', #10338, #6311 ) ;
#22978=AXIS2_PLACEMENT_3D ( 'NONE', #9205, #19691, #14134 ) ;
#22988=CARTESIAN_POINT ( 'NONE',  ( 21.09785597605719332, 48.06454579224779877, 47.04930799450051637 ) ) ;
#23024=ORIENTED_EDGE ( 'NONE', *, *, #14839, .F. ) ;
#23030=AXIS2_PLACEMENT_3D ( 'NONE', #17360, #15991, #20911 ) ;
#23039=EDGE_CURVE ( 'NONE', #16313, #31740, #21418, .T. ) ;
#23078=DIRECTION ( 'NONE',  ( 0.000000000000000000, 0.000000000000000000, 1.000000000000000000 ) ) ;
#23086=FACE_OUTER_BOUND ( 'NONE', #6379, .T. ) ;
#23087=AXIS2_PLACEMENT_3D ( 'NONE', #24574, #14410, #29513 ) ;
#23094=VECTOR ( 'NONE', #31530, 1000.000000000000000 ) ;
#23111=AXIS2_PLACEMENT_3D ( 'NONE', #15530, #20618, #25542 ) ;
#23116=CARTESIAN_POINT ( 'NONE',  ( 21.09785597605719332, 30.56454579224779522, 64.04930799450050927 ) ) ;
#23121=ORIENTED_EDGE ( 'NONE', *, *, #6636, .T. ) ;
#23123=CIRCLE ( 'NONE', #8972, 13.20000000000000284 ) ;
#23155=CONICAL_SURFACE ( 'NONE', #6918, 31.29999999999997939, 0.7853981633974482790 ) ;
#23204=EDGE_CURVE ( 'NONE', #28894, #30447, #28046, .T. ) ;
#23242=LINE ( 'NONE', #13555, #11498 ) ;
#23254=CARTESIAN_POINT ( 'NONE',  ( 21.09785597605719332, 43.56454579224774193, 47.04930799450051637 ) ) ;
#23260=CARTESIAN_POINT ( 'NONE',  ( 21.09785597605719332, 43.56454579224774193, 47.04930799450051637 ) ) ;
#23292=AXIS2_PLACEMENT_3D ( 'NONE', #20044, #12515, #9556 ) ;
#23306=DIRECTION ( 'NONE',  ( 0.000000000000000000, -1.000000000000000000, 0.000000000000000000 ) ) ;
#23316=DIRECTION ( 'NONE',  ( -0.000000000000000000, -1.000000000000000000, -0.000000000000000000 ) ) ;
#23353=DIRECTION ( 'NONE',  ( 0.000000000000000000, 1.000000000000000000, 0.000000000000000000 ) ) ;
#23359=CONICAL_SURFACE ( 'NONE', #19669, 19.04889477833696176, 0.8552113334772211140 ) ;
#23380=DIRECTION ( 'NONE',  ( -0.000000000000000000, 1.000000000000000000, -0.000000000000000000 ) ) ;
#23389=EDGE_CURVE ( 'NONE', #32160, #4198, #21439, .T. ) ;
#23412=DIRECTION ( 'NONE',  ( 0.000000000000000000, 0.000000000000000000, -1.000000000000000000 ) ) ;
#23498=CARTESIAN_POINT ( 'NONE',  ( 21.09785597605719332, 43.75535478762431296, 18.03093517794834000 ) ) ;
#23524=FACE_OUTER_BOUND ( 'NONE', #28310, .T. ) ;
#23525=SURFACE_STYLE_FILL_AREA ( #1516 ) ;
#23534=DIRECTION ( 'NONE',  ( 0.000000000000000000, -1.000000000000000000, 0.000000000000000000 ) ) ;
#23536=VERTEX_POINT ( 'NONE', #25539 ) ;
#23538=CARTESIAN_POINT ( 'NONE',  ( 21.09785597605719687, 43.56454579224774193, 77.04930799450052348 ) ) ;
#23584=ORIENTED_EDGE ( 'NONE', *, *, #6710, .T. ) ;
#23606=MECHANICAL_DESIGN_GEOMETRIC_PRESENTATION_REPRESENTATION('',(#1066),#20473);
#23613=DIRECTION ( 'NONE',  ( -0.000000000000000000, -1.000000000000000000, -0.000000000000000000 ) ) ;
#23615=EDGE_CURVE ( 'NONE', #24681, #7753, #23242, .T. ) ;
#23654=EDGE_LOOP ( 'NONE', ( #20128, #26084, #25441, #2626 ) ) ;
#23668=EDGE_CURVE ( 'NONE', #3952, #12727, #32481, .T. ) ;
#23672=CIRCLE ( 'NONE', #24708, 22.50178251985260758 ) ;
#23695=VERTEX_POINT ( 'NONE', #1389 ) ;
#23703=DIRECTION ( 'NONE',  ( 0.000000000000000000, 0.000000000000000000, 1.000000000000000000 ) ) ;
#23709=ADVANCED_FACE ( 'NONE', ( #6322 ), #11019, .F. ) ;
#23712=EDGE_CURVE ( 'NONE', #6391, #6454, #19385, .T. ) ;
#23749=DIRECTION ( 'NONE',  ( 0.000000000000000000, 1.000000000000000000, 0.000000000000000000 ) ) ;
#23756=DIRECTION ( 'NONE',  ( 0.000000000000000000, 0.000000000000000000, 1.000000000000000000 ) ) ;
#23803=VERTEX_POINT ( 'NONE', #17788 ) ;
#23811=ORIENTED_EDGE ( 'NONE', *, *, #30183, .F. ) ;
#23822=AXIS2_PLACEMENT_3D ( 'NONE', #24642, #4459, #4295 ) ;
#23831=DIRECTION ( 'NONE',  ( 0.000000000000000000, -1.000000000000000000, 0.000000000000000000 ) ) ;
#23878=ORIENTED_EDGE ( 'NONE', *, *, #8535, .F. ) ;
#23890=EDGE_CURVE ( 'NONE', #6391, #5554, #2699, .T. ) ;
#23936=EDGE_CURVE ( 'NONE', #15830, #7227, #4840, .T. ) ;
#23999=SURFACE_SIDE_STYLE ('',( #23525 ) ) ;
#24024=VECTOR ( 'NONE', #13874, 1000.000000000000000 ) ;
#24038=DIRECTION ( 'NONE',  ( 0.000000000000000000, 1.000000000000000000, 0.000000000000000000 ) ) ;
#24045=CYLINDRICAL_SURFACE ( 'NONE', #31545, 13.00000000000000533 ) ;
#24065=ADVANCED_FACE ( 'NONE', ( #18110 ), #28295, .T. ) ;
#24070=DIRECTION ( 'NONE',  ( 0.000000000000000000, -0.000000000000000000, -1.000000000000000000 ) ) ;
#24104=ORIENTED_EDGE ( 'NONE', *, *, #18651, .F. ) ;
#24106=AXIS2_PLACEMENT_3D ( 'NONE', #9648, #17517, #2580 ) ;
#24181=AXIS2_PLACEMENT_3D ( 'NONE', #3220, #15536, #18474 ) ;
#24205=DIRECTION ( 'NONE',  ( -0.000000000000000000, -1.000000000000000000, -0.000000000000000000 ) ) ;
#24214=CARTESIAN_POINT ( 'NONE',  ( 21.09785597605719332, 25.56454579224779877, 47.04930799450051637 ) ) ;
#24220=DIRECTION ( 'NONE',  ( 0.000000000000000000, 0.000000000000000000, 1.000000000000000000 ) ) ;
#24247=CARTESIAN_POINT ( 'NONE',  ( 21.09785597605719687, 30.56454579224779522, 30.04930799450051282 ) ) ;
#24278=EDGE_CURVE ( 'NONE', #28333, #257, #19414, .T. ) ;
#24333=DIRECTION ( 'NONE',  ( -0.000000000000000000, -1.000000000000000000, -0.000000000000000000 ) ) ;
#24361=PLANE ( 'NONE',  #13930 ) ;
#24374=( NAMED_UNIT ( * ) SI_UNIT ( $, .STERADIAN. ) SOLID_ANGLE_UNIT ( ) );
#24395=ORIENTED_EDGE ( 'NONE', *, *, #11522, .T. ) ;
#24398=CARTESIAN_POINT ( 'NONE',  ( 21.09785597605719332, 25.56454579224779167, 47.04930799450051637 ) ) ;
#24406=CARTESIAN_POINT ( 'NONE',  ( 21.09785597605719332, 40.56454579224780588, 59.54930799450053769 ) ) ;
#24421=AXIS2_PLACEMENT_3D ( 'NONE', #8543, #18533, #18855 ) ;
#24449=CARTESIAN_POINT ( 'NONE',  ( 21.09785597605719332, 44.06454579224779877, 47.04930799450051637 ) ) ;
#24450=DIRECTION ( 'NONE',  ( 0.000000000000000000, -1.000000000000000000, 0.000000000000000000 ) ) ;
#24517=CARTESIAN_POINT ( 'NONE',  ( 21.09785597605719687, 40.56454579224780588, 17.04930799450051637 ) ) ;
#24524=AXIS2_PLACEMENT_3D ( 'NONE', #19070, #6130, #15981 ) ;
#24533=DIRECTION ( 'NONE',  ( 0.000000000000000000, 0.000000000000000000, 1.000000000000000000 ) ) ;
#24574=CARTESIAN_POINT ( 'NONE',  ( 21.09785597605719332, 25.76454579224776964, 47.04930799450051637 ) ) ;
#24575=CARTESIAN_POINT ( 'NONE',  ( 21.09785597605719332, 25.56454579224779167, 78.34930799450054906 ) ) ;
#24611=ORIENTED_EDGE ( 'NONE', *, *, #8848, .T. ) ;
#24642=CARTESIAN_POINT ( 'NONE',  ( 21.09785597605719332, 45.28940914544685370, 69.74790822305027405 ) ) ;
#24646=ORIENTED_EDGE ( 'NONE', *, *, #2924, .F. ) ;
#24649=ADVANCED_FACE ( 'NONE', ( #21778 ), #1601, .T. ) ;
#24669=CARTESIAN_POINT ( 'NONE',  ( 21.09785597605719687, 48.06454579224779877, 66.09820277283748169 ) ) ;
#24673=ORIENTED_EDGE ( 'NONE', *, *, #11571, .T. ) ;
#24681=VERTEX_POINT ( 'NONE', #24247 ) ;
#24701=ORIENTED_EDGE ( 'NONE', *, *, #32357, .F. ) ;
#24708=AXIS2_PLACEMENT_3D ( 'NONE', #11420, #1408, #11591 ) ;
#24712=ORIENTED_EDGE ( 'NONE', *, *, #14359, .F. ) ;
#24778=ORIENTED_EDGE ( 'NONE', *, *, #29715, .T. ) ;
#24793=TOROIDAL_SURFACE ( 'NONE', #29532, 22.69860022854976123, 0.2999999999999999889 ) ;
#24813=LINE ( 'NONE', #29910, #15970 ) ;
#24842=DIRECTION ( 'NONE',  ( -0.000000000000000000, -1.000000000000000000, -0.000000000000000000 ) ) ;
#24873=CONICAL_SURFACE ( 'NONE', #19624, 13.20000000000000995, 0.7853981633974612686 ) ;
#24883=VERTEX_POINT ( 'NONE', #14360 ) ;
#24892=DIRECTION ( 'NONE',  ( 0.000000000000000000, 0.000000000000000000, 1.000000000000000000 ) ) ;
#24906=ADVANCED_FACE ( 'NONE', ( #7291 ), #11863, .T. ) ;
#24920=CYLINDRICAL_SURFACE ( 'NONE', #6653, 2.500000000000002220 ) ;
#24928=ORIENTED_EDGE ( 'NONE', *, *, #31145, .F. ) ;
#24947=CIRCLE ( 'NONE', #1877, 13.00000000000000533 ) ;
#24967=DIRECTION ( 'NONE',  ( 0.000000000000000000, 0.000000000000000000, 1.000000000000000000 ) ) ;
#24977=CARTESIAN_POINT ( 'NONE',  ( 21.09785597605719687, 30.56454579224779522, 78.54930799450052348 ) ) ;
#25003=DIRECTION ( 'NONE',  ( 0.000000000000000000, 0.000000000000000000, 1.000000000000000000 ) ) ;
#25032=DIRECTION ( 'NONE',  ( 0.000000000000000000, 0.000000000000000000, 1.000000000000000000 ) ) ;
#25047=EDGE_CURVE ( 'NONE', #23695, #1790, #23123, .T. ) ;
#25077=AXIS2_PLACEMENT_3D ( 'NONE', #21191, #23353, #16114 ) ;
#25192=DIRECTION ( 'NONE',  ( 0.000000000000000000, 0.000000000000000000, -1.000000000000000000 ) ) ;
#25209=AXIS2_PLACEMENT_3D ( 'NONE', #3047, #13084, #23078 ) ;
#25217=DIRECTION ( 'NONE',  ( 8.659560562355045024E-17, -0.7071067811865383579, 0.7071067811865566766 ) ) ;
#25266=CARTESIAN_POINT ( 'NONE',  ( 21.09785597605719332, 25.56454579224779877, 59.04930799450051637 ) ) ;
#25267=VERTEX_POINT ( 'NONE', #10138 ) ;
#25282=EDGE_CURVE ( 'NONE', #12063, #13560, #18932, .T. ) ;
#25327=ORIENTED_EDGE ( 'NONE', *, *, #27999, .F. ) ;
#25328=ORIENTED_EDGE ( 'NONE', *, *, #1816, .T. ) ;
#25338=EDGE_LOOP ( 'NONE', ( #1060, #638, #11870, #30556 ) ) ;
#25342=CARTESIAN_POINT ( 'NONE',  ( 21.09785597605719332, 25.56454579224779167, 73.04930799450052348 ) ) ;
#25367=TOROIDAL_SURFACE ( 'NONE', #16421, 22.69860022854976123, 0.2999999999999999889 ) ;
#25382=VERTEX_POINT ( 'NONE', #10944 ) ;
#25389=ADVANCED_FACE ( 'NONE', ( #5209 ), #25549, .F. ) ;
#25399=ORIENTED_EDGE ( 'NONE', *, *, #4149, .T. ) ;
#25410=TOROIDAL_SURFACE ( 'NONE', #3917, 18.86195243859455672, 0.5000000000000000000 ) ;
#25415=ADVANCED_FACE ( 'NONE', ( #23086 ), #25767, .T. ) ;
#25429=DIRECTION ( 'NONE',  ( 0.000000000000000000, 0.000000000000000000, 1.000000000000000000 ) ) ;
#25436=EDGE_LOOP ( 'NONE', ( #18331, #6113 ) ) ;
#25441=ORIENTED_EDGE ( 'NONE', *, *, #2432, .T. ) ;
#25444=APPLICATION_CONTEXT ( 'automotive_design' ) ;
#25453=VERTEX_POINT ( 'NONE', #31131 ) ;
#25454=DIRECTION ( 'NONE',  ( 0.000000000000000000, 0.000000000000000000, -1.000000000000000000 ) ) ;
#25458=ADVANCED_FACE ( 'NONE', ( #8641 ), #24045, .F. ) ;
#25471=ADVANCED_FACE ( 'NONE', ( #11265 ), #98, .T. ) ;
#25539=CARTESIAN_POINT ( 'NONE',  ( -4.902144023942810236, 30.56454579224779522, 44.54930799450042400 ) ) ;
#25542=DIRECTION ( 'NONE',  ( 0.000000000000000000, 0.000000000000000000, 1.000000000000000000 ) ) ;
#25549=CYLINDRICAL_SURFACE ( 'NONE', #6370, 2.499999999999998668 ) ;
#25551=DIRECTION ( 'NONE',  ( 0.000000000000000000, 0.000000000000000000, 1.000000000000000000 ) ) ;
#25563=UNCERTAINTY_MEASURE_WITH_UNIT (LENGTH_MEASURE( 1.000000000000000082E-05 ), #30924, 'distance_accuracy_value', 'NONE');
#25572=ORIENTED_EDGE ( 'NONE', *, *, #23204, .F. ) ;
#25575=DIRECTION ( 'NONE',  ( -0.000000000000000000, 1.000000000000000000, -0.000000000000000000 ) ) ;
#25579=ORIENTED_EDGE ( 'NONE', *, *, #31344, .F. ) ;
#25593=FACE_OUTER_BOUND ( 'NONE', #31472, .T. ) ;
#25600=CARTESIAN_POINT ( 'NONE',  ( 21.09785597605719332, 28.56454579224779877, 46.64306900320794114 ) ) ;
#25602=DIRECTION ( 'NONE',  ( 0.000000000000000000, 0.000000000000000000, 1.000000000000000000 ) ) ;
#25609=ADVANCED_FACE ( 'NONE', ( #1887 ), #4848, .T. ) ;
#25620=DIRECTION ( 'NONE',  ( -0.000000000000000000, -1.000000000000000000, -0.000000000000000000 ) ) ;
#25644=EDGE_CURVE ( 'NONE', #11408, #30811, #12168, .T. ) ;
#25711=ORIENTED_EDGE ( 'NONE', *, *, #25282, .T. ) ;
#25728=ORIENTED_EDGE ( 'NONE', *, *, #28888, .T. ) ;
#25731=LINE ( 'NONE', #21269, #19540 ) ;
#25733=ORIENTED_EDGE ( 'NONE', *, *, #26797, .F. ) ;
#25739=AXIS2_PLACEMENT_3D ( 'NONE', #17662, #28011, #8155 ) ;
#25741=AXIS2_PLACEMENT_3D ( 'NONE', #4318, #8914, #3991 ) ;
#25767=CONICAL_SURFACE ( 'NONE', #30501, 30.00000000000000000, 1.378810109075523149 ) ;
#25786=LINE ( 'NONE', #15301, #47 ) ;
#25801=VERTEX_POINT ( 'NONE', #8122 ) ;
#25856=ADVANCED_FACE ( 'NONE', ( #3987 ), #31571, .F. ) ;
#25859=ORIENTED_EDGE ( 'NONE', *, *, #1801, .T. ) ;
#25869=CARTESIAN_POINT ( 'NONE',  ( 21.09785597605719332, 25.56454579224779167, 21.04930799450051282 ) ) ;
#25892=ORIENTED_EDGE ( 'NONE', *, *, #24278, .F. ) ;
#25897=EDGE_CURVE ( 'NONE', #13560, #12063, #12507, .T. ) ;
#25964=VERTEX_POINT ( 'NONE', #13692 ) ;
#25988=CIRCLE ( 'NONE', #11312, 11.79999999999997762 ) ;
#26025=ORIENTED_EDGE ( 'NONE', *, *, #2953, .F. ) ;
#26031=ORIENTED_EDGE ( 'NONE', *, *, #6636, .F. ) ;
#26084=ORIENTED_EDGE ( 'NONE', *, *, #18554, .F. ) ;
#26088=FACE_BOUND ( 'NONE', #18686, .T. ) ;
#26113=ORIENTED_EDGE ( 'NONE', *, *, #29715, .F. ) ;
#26132=LINE ( 'NONE', #8421, #9628 ) ;
#26137=VECTOR ( 'NONE', #11556, 1000.000000000000227 ) ;
#26163=EDGE_LOOP ( 'NONE', ( #15460, #14348, #18285, #13794 ) ) ;
#26187=CARTESIAN_POINT ( 'NONE',  ( 21.09785597605719332, 25.56454579224779167, 47.04930799450051637 ) ) ;
#26251=ORIENTED_EDGE ( 'NONE', *, *, #12776, .T. ) ;
#26260=LINE ( 'NONE', #3769, #13654 ) ;
#26272=DIRECTION ( 'NONE',  ( 0.000000000000000000, 0.000000000000000000, -1.000000000000000000 ) ) ;
#26310=CARTESIAN_POINT ( 'NONE',  ( 21.09785597605719332, 25.76454579224781227, 59.04930799450051637 ) ) ;
#26323=ORIENTED_EDGE ( 'NONE', *, *, #30183, .T. ) ;
#26357=ORIENTED_EDGE ( 'NONE', *, *, #12776, .F. ) ;
#26380=CARTESIAN_POINT ( 'NONE',  ( 47.09785597605719687, 30.56554579224779644, 44.54930799450078638 ) ) ;
#26383=AXIS2_PLACEMENT_3D ( 'NONE', #12615, #22430, #17353 ) ;
#26398=DIRECTION ( 'NONE',  ( 0.000000000000000000, 0.000000000000000000, -1.000000000000000000 ) ) ;
#26403=DIRECTION ( 'NONE',  ( 0.000000000000000000, -1.000000000000000000, 0.000000000000000000 ) ) ;
#26413=EDGE_CURVE ( 'NONE', #25382, #8568, #12531, .T. ) ;
#26440=DIRECTION ( 'NONE',  ( 0.000000000000000000, 0.000000000000000000, 1.000000000000000000 ) ) ;
#26470=ADVANCED_BREP_SHAPE_REPRESENTATION ( '', ( #12454, #8172 ), #9736 ) ;
#26471=SURFACE_STYLE_USAGE ( .BOTH. , #23999 ) ;
#26495=ORIENTED_EDGE ( 'NONE', *, *, #27239, .F. ) ;
#26500=DIRECTION ( 'NONE',  ( 0.000000000000000000, 0.000000000000000000, 1.000000000000000000 ) ) ;
#26542=CARTESIAN_POINT ( 'NONE',  ( 21.09785597605719332, 40.06454579224778456, 35.04930799450050927 ) ) ;
#26588=PRODUCT_DEFINITION_SHAPE ( 'NONE', 'NONE',  #8108 ) ;
#26590=DIRECTION ( 'NONE',  ( -0.000000000000000000, -1.000000000000000000, -0.000000000000000000 ) ) ;
#26609=CIRCLE ( 'NONE', #11920, 32.50000000000000000 ) ;
#26617=VERTEX_POINT ( 'NONE', #11310 ) ;
#26637=CARTESIAN_POINT ( 'NONE',  ( 21.09785597605719332, 40.56454579224779877, 79.54930799450052348 ) ) ;
#26658=EDGE_CURVE ( 'NONE', #1564, #28978, #21341, .T. ) ;
#26678=( LENGTH_UNIT ( ) NAMED_UNIT ( * ) SI_UNIT ( .MILLI., .METRE. ) );
#26696=EDGE_CURVE ( 'NONE', #20780, #20710, #7216, .T. ) ;
#26698=CARTESIAN_POINT ( 'NONE',  ( 21.09785597605719332, 30.56454579224779522, 47.04930799450051637 ) ) ;
#26703=ORIENTED_EDGE ( 'NONE', *, *, #16298, .T. ) ;
#26712=AXIS2_PLACEMENT_3D ( 'NONE', #8609, #16142, #20594 ) ;
#26743=DIRECTION ( 'NONE',  ( 0.000000000000000000, 0.000000000000000000, 1.000000000000000000 ) ) ;
#26751=DIRECTION ( 'NONE',  ( 0.000000000000000000, 0.000000000000000000, 1.000000000000000000 ) ) ;
#26757=CARTESIAN_POINT ( 'NONE',  ( 21.09785597605719332, 40.56454579224780588, 34.54930799450048795 ) ) ;
#26769=DIRECTION ( 'NONE',  ( -0.000000000000000000, -1.000000000000000000, -0.000000000000000000 ) ) ;
#26772=CONICAL_SURFACE ( 'NONE', #45, 30.00000000000000000, 0.5934119456780768687 ) ;
#26778=CARTESIAN_POINT ( 'NONE',  ( -4.902144023942810236, 30.56454579224779522, 47.04930799450042400 ) ) ;
#26795=EDGE_CURVE ( 'NONE', #25801, #20484, #26609, .T. ) ;
#26796=DIRECTION ( 'NONE',  ( 0.000000000000000000, 1.000000000000000000, 0.000000000000000000 ) ) ;
#26797=EDGE_CURVE ( 'NONE', #1790, #23695, #16109, .T. ) ;
#26798=ORIENTED_EDGE ( 'NONE', *, *, #26658, .F. ) ;
#26803=CARTESIAN_POINT ( 'NONE',  ( 47.09785597605719687, 30.56454579224779522, 47.04930799450078638 ) ) ;
#26820=EDGE_LOOP ( 'NONE', ( #21297, #30879, #9588, #20559 ) ) ;
#26827=ORIENTED_EDGE ( 'NONE', *, *, #23204, .T. ) ;
#26828=FACE_OUTER_BOUND ( 'NONE', #27353, .T. ) ;
#26847=LINE ( 'NONE', #29478, #13834 ) ;
#26884=CARTESIAN_POINT ( 'NONE',  ( -4.902144023942810236, 30.56454579224779522, 47.04930799450042400 ) ) ;
#26894=ORIENTED_EDGE ( 'NONE', *, *, #14409, .T. ) ;
#26902=EDGE_CURVE ( 'NONE', #22757, #28878, #10762, .T. ) ;
#26920=CARTESIAN_POINT ( 'NONE',  ( 21.09785597605719332, 25.56454579224779877, 47.04930799450051637 ) ) ;
#26946=CARTESIAN_POINT ( 'NONE',  ( 21.09785597605719332, 30.56454579224779522, 47.04930799450051637 ) ) ;
#26964=AXIS2_PLACEMENT_3D ( 'NONE', #32170, #17216, #26751 ) ;
#26984=EDGE_LOOP ( 'NONE', ( #14996, #1975, #24395, #25327 ) ) ;
#27003=DIRECTION ( 'NONE',  ( 0.000000000000000000, -0.000000000000000000, 1.000000000000000000 ) ) ;
#27089=DIRECTION ( 'NONE',  ( 0.000000000000000000, -0.000000000000000000, -1.000000000000000000 ) ) ;
#27139=ORIENTED_EDGE ( 'NONE', *, *, #29293, .T. ) ;
#27170=CONICAL_SURFACE ( 'NONE', #25077, 0.9999999999999731326, 0.4537856055185219284 ) ;
#27183=CARTESIAN_POINT ( 'NONE',  ( 47.09785597605719687, 25.56454579224779167, 49.54930799450078638 ) ) ;
#27239=EDGE_CURVE ( 'NONE', #7227, #27529, #5272, .T. ) ;
#27316=EDGE_CURVE ( 'NONE', #22063, #25801, #29441, .T. ) ;
#27341=VECTOR ( 'NONE', #3872, 1000.000000000000000 ) ;
#27353=EDGE_LOOP ( 'NONE', ( #23121, #27139 ) ) ;
#27435=LINE ( 'NONE', #12511, #27613 ) ;
#27489=DIRECTION ( 'NONE',  ( 0.000000000000000000, 0.000000000000000000, 1.000000000000000000 ) ) ;
#27506=CARTESIAN_POINT ( 'NONE',  ( 21.09785597605719332, 48.06454579224779877, 28.00041321616355461 ) ) ;
#27529=VERTEX_POINT ( 'NONE', #31543 ) ;
#27542=CARTESIAN_POINT ( 'NONE',  ( 21.09785597605719332, 30.56554579224779644, 73.04930799450052348 ) ) ;
#27576=ORIENTED_EDGE ( 'NONE', *, *, #10967, .T. ) ;
#27613=VECTOR ( 'NONE', #10042, 1000.000000000000000 ) ;
#27618=ORIENTED_EDGE ( 'NONE', *, *, #18651, .T. ) ;
#27619=DIRECTION ( 'NONE',  ( 0.000000000000000000, 0.000000000000000000, -1.000000000000000000 ) ) ;
#27636=ADVANCED_FACE ( 'NONE', ( #21991 ), #26772, .T. ) ;
#27685=ORIENTED_EDGE ( 'NONE', *, *, #24278, .T. ) ;
#27718=CIRCLE ( 'NONE', #17238, 12.00000000000000355 ) ;
#27739=CARTESIAN_POINT ( 'NONE',  ( -4.902144023942810236, 30.56454579224779522, 49.54930799450042400 ) ) ;
#27764=VECTOR ( 'NONE', #12729, 1000.000000000000000 ) ;
#27767=CYLINDRICAL_SURFACE ( 'NONE', #10638, 12.00000000000000355 ) ;
#27810=VECTOR ( 'NONE', #28258, 1000.000000000000000 ) ;
#27819=DIRECTION ( 'NONE',  ( 0.000000000000000000, 0.000000000000000000, 1.000000000000000000 ) ) ;
#27833=EDGE_LOOP ( 'NONE', ( #25711, #27881, #30582, #15378 ) ) ;
#27854=DIRECTION ( 'NONE',  ( 0.000000000000000000, 0.000000000000000000, -1.000000000000000000 ) ) ;
#27865=DIRECTION ( 'NONE',  ( 0.000000000000000000, 0.000000000000000000, -1.000000000000000000 ) ) ;
#27880=CIRCLE ( 'NONE', #29446, 0.4062389912925720714 ) ;
#27881=ORIENTED_EDGE ( 'NONE', *, *, #12224, .T. ) ;
#27930=DIRECTION ( 'NONE',  ( 1.000000000000000000, 0.000000000000000000, 2.775557561562892534E-15 ) ) ;
#27933=VECTOR ( 'NONE', #21294, 1000.000000000000000 ) ;
#27973=CARTESIAN_POINT ( 'NONE',  ( 21.09785597605719332, 30.56554579224779644, 75.54930799450052348 ) ) ;
#27982=DIRECTION ( 'NONE',  ( -0.000000000000000000, -1.000000000000000000, -0.000000000000000000 ) ) ;
#27999=EDGE_CURVE ( 'NONE', #30811, #11408, #17790, .T. ) ;
#28011=DIRECTION ( 'NONE',  ( -0.000000000000000000, 1.000000000000000000, -0.000000000000000000 ) ) ;
#28036=CYLINDRICAL_SURFACE ( 'NONE', #2068, 2.500000000000002220 ) ;
#28040=CIRCLE ( 'NONE', #23822, 0.2999999999999947153 ) ;
#28046=LINE ( 'NONE', #23116, #12002 ) ;
#28080=MECHANICAL_DESIGN_GEOMETRIC_PRESENTATION_REPRESENTATION('',(#14473),#13926);
#28090=ORIENTED_EDGE ( 'NONE', *, *, #22252, .T. ) ;
#28142=ORIENTED_EDGE ( 'NONE', *, *, #8535, .T. ) ;
#28175=ORIENTED_EDGE ( 'NONE', *, *, #22438, .T. ) ;
#28206=ADVANCED_FACE ( 'NONE', ( #17687 ), #28036, .F. ) ;
#28258=DIRECTION ( 'NONE',  ( -0.000000000000000000, 1.000000000000000000, 0.000000000000000000 ) ) ;
#28292=CIRCLE ( 'NONE', #17813, 31.30000000000002913 ) ;
#28295=CYLINDRICAL_SURFACE ( 'NONE', #28330, 12.00000000000000355 ) ;
#28298=PRESENTATION_STYLE_ASSIGNMENT (( #26471 ) ) ;
#28310=EDGE_LOOP ( 'NONE', ( #691, #21960, #2879, #18548 ) ) ;
#28330=AXIS2_PLACEMENT_3D ( 'NONE', #3168, #15818, #14165 ) ;
#28333=VERTEX_POINT ( 'NONE', #6034 ) ;
#28341=CYLINDRICAL_SURFACE ( 'NONE', #11282, 32.50000000000000711 ) ;
#28380=ORIENTED_EDGE ( 'NONE', *, *, #26413, .T. ) ;
#28395=CARTESIAN_POINT ( 'NONE',  ( 21.09785597605719332, 30.56454579224779522, 47.04930799450051637 ) ) ;
#28444=DIRECTION ( 'NONE',  ( 0.000000000000000000, -0.7071067811865474617, -0.7071067811865474617 ) ) ;
#28490=ORIENTED_EDGE ( 'NONE', *, *, #21653, .F. ) ;
#28497=LINE ( 'NONE', #8474, #3719 ) ;
#28502=DIRECTION ( 'NONE',  ( 0.000000000000000000, 0.000000000000000000, 1.000000000000000000 ) ) ;
#28503=CARTESIAN_POINT ( 'NONE',  ( 21.09785597605719332, 48.06454579224779877, 47.04930799450051637 ) ) ;
#28505=VERTEX_POINT ( 'NONE', #8741 ) ;
#28506=DIRECTION ( 'NONE',  ( -0.000000000000000000, 1.000000000000000000, -0.000000000000000000 ) ) ;
#28516=DIRECTION ( 'NONE',  ( 0.000000000000000000, 0.000000000000000000, -1.000000000000000000 ) ) ;
#28555=DIRECTION ( 'NONE',  ( -0.000000000000000000, -1.000000000000000000, -0.000000000000000000 ) ) ;
#28579=EDGE_CURVE ( 'NONE', #24883, #20484, #13684, .T. ) ;
#28707=EDGE_LOOP ( 'NONE', ( #24928, #16759, #31286, #29527 ) ) ;
#28717=AXIS2_PLACEMENT_3D ( 'NONE', #6877, #3922, #29192 ) ;
#28733=DIRECTION ( 'NONE',  ( 0.000000000000000000, 0.000000000000000000, 1.000000000000000000 ) ) ;
#28736=EDGE_LOOP ( 'NONE', ( #26113, #3615, #16397, #8396 ) ) ;
#28764=ORIENTED_EDGE ( 'NONE', *, *, #14421, .T. ) ;
#28770=( NAMED_UNIT ( * ) SI_UNIT ( $, .STERADIAN. ) SOLID_ANGLE_UNIT ( ) );
#28838=AXIS2_PLACEMENT_3D ( 'NONE', #17111, #9251, #4650 ) ;
#28878=VERTEX_POINT ( 'NONE', #31690 ) ;
#28888=EDGE_CURVE ( 'NONE', #5554, #19454, #30432, .T. ) ;
#28892=DIRECTION ( 'NONE',  ( -0.000000000000000000, -1.000000000000000000, -0.000000000000000000 ) ) ;
#28894=VERTEX_POINT ( 'NONE', #6902 ) ;
#28915=DIRECTION ( 'NONE',  ( 0.000000000000000000, -1.000000000000000000, 0.000000000000000000 ) ) ;
#28932=FACE_OUTER_BOUND ( 'NONE', #14566, .T. ) ;
#28935=EDGE_CURVE ( 'NONE', #8568, #30811, #11666, .T. ) ;
#28958=CARTESIAN_POINT ( 'NONE',  ( 21.09785597605719687, 45.06299627138002251, 69.55109051435312040 ) ) ;
#28960=ORIENTED_EDGE ( 'NONE', *, *, #29948, .T. ) ;
#28978=VERTEX_POINT ( 'NONE', #26757 ) ;
#28984=ADVANCED_FACE ( 'NONE', ( #7061 ), #11831, .T. ) ;
#28990=DIRECTION ( 'NONE',  ( 0.000000000000000000, 0.000000000000000000, 1.000000000000000000 ) ) ;
#28998=VECTOR ( 'NONE', #18355, 1000.000000000000000 ) ;
#29054=ORIENTED_EDGE ( 'NONE', *, *, #29059, .T. ) ;
#29059=EDGE_CURVE ( 'NONE', #5208, #22400, #22956, .T. ) ;
#29065=CYLINDRICAL_SURFACE ( 'NONE', #13507, 32.50000000000000711 ) ;
#29103=AXIS2_PLACEMENT_3D ( 'NONE', #25869, #3379, #28502 ) ;
#29111=CARTESIAN_POINT ( 'NONE',  ( 21.09785597605719332, 42.30003263981368633, 47.04930799450051637 ) ) ;
#29161=EDGE_CURVE ( 'NONE', #30996, #19482, #13706, .T. ) ;
#29165=ORIENTED_EDGE ( 'NONE', *, *, #1779, .T. ) ;
#29192=DIRECTION ( 'NONE',  ( 0.000000000000000000, 0.000000000000000000, -1.000000000000000000 ) ) ;
#29198=CIRCLE ( 'NONE', #15061, 30.00000000000000711 ) ;
#29254=CARTESIAN_POINT ( 'NONE',  ( 21.09785597605719332, 48.06454579224779877, 47.04930799450051637 ) ) ;
#29290=CARTESIAN_POINT ( 'NONE',  ( 21.09785597605719332, 30.56454579224779522, 47.04930799450051637 ) ) ;
#29293=EDGE_CURVE ( 'NONE', #22063, #24883, #17334, .T. ) ;
#29295=DIRECTION ( 'NONE',  ( -0.000000000000000000, -1.000000000000000000, 0.000000000000000000 ) ) ;
#29300=DIRECTION ( 'NONE',  ( 0.000000000000000000, 1.000000000000000000, 0.000000000000000000 ) ) ;
#29326=FACE_BOUND ( 'NONE', #18664, .T. ) ;
#29362=CIRCLE ( 'NONE', #3680, 2.499999999999998668 ) ;
#29380=ORIENTED_EDGE ( 'NONE', *, *, #22300, .F. ) ;
#29434=EDGE_CURVE ( 'NONE', #18274, #30996, #18896, .T. ) ;
#29441=LINE ( 'NONE', #5789, #4211 ) ;
#29446=AXIS2_PLACEMENT_3D ( 'NONE', #32096, #5338, #25192 ) ;
#29463=FACE_BOUND ( 'NONE', #20238, .T. ) ;
#29478=CARTESIAN_POINT ( 'NONE',  ( 21.09785597605719332, 25.56454579224779877, 58.84930799450049221 ) ) ;
#29494=LINE ( 'NONE', #18971, #19260 ) ;
#29508=CARTESIAN_POINT ( 'NONE',  ( 21.09785597605719332, 40.56454579224780588, 47.04930799450051637 ) ) ;
#29513=DIRECTION ( 'NONE',  ( 0.000000000000000000, 0.000000000000000000, 1.000000000000000000 ) ) ;
#29527=ORIENTED_EDGE ( 'NONE', *, *, #3988, .T. ) ;
#29532=AXIS2_PLACEMENT_3D ( 'NONE', #19140, #4225, #23756 ) ;
#29538=DIRECTION ( 'NONE',  ( 0.000000000000000000, 0.000000000000000000, -1.000000000000000000 ) ) ;
#29617=ADVANCED_FACE ( 'NONE', ( #13266 ), #8976, .T. ) ;
#29625=DIRECTION ( 'NONE',  ( 0.000000000000000000, -1.000000000000000000, 0.000000000000000000 ) ) ;
#29638=ORIENTED_EDGE ( 'NONE', *, *, #13628, .F. ) ;
#29648=EDGE_CURVE ( 'NONE', #5195, #28505, #17890, .T. ) ;
#29649=ADVANCED_FACE ( 'NONE', ( #31614 ), #13722, .T. ) ;
#29655=DIRECTION ( 'NONE',  ( 0.000000000000000000, 0.000000000000000000, 1.000000000000000000 ) ) ;
#29661=CARTESIAN_POINT ( 'NONE',  ( 21.09785597605719332, 30.36454579224779238, 60.04930799450051637 ) ) ;
#29715=EDGE_CURVE ( 'NONE', #18274, #13855, #23672, .T. ) ;
#29733=ORIENTED_EDGE ( 'NONE', *, *, #13031, .F. ) ;
#29744=PLANE ( 'NONE',  #2325 ) ;
#29746=DIRECTION ( 'NONE',  ( -0.000000000000000000, -1.000000000000000000, 0.000000000000000000 ) ) ;
#29775=ORIENTED_EDGE ( 'NONE', *, *, #25047, .T. ) ;
#29807=ADVANCED_FACE ( 'NONE', ( #17311 ), #3727, .T. ) ;
#29829=EDGE_CURVE ( 'NONE', #20710, #20780, #21549, .T. ) ;
#29898=VECTOR ( 'NONE', #10742, 1000.000000000000000 ) ;
#29910=CARTESIAN_POINT ( 'NONE',  ( 21.09785597605719332, 40.06454579224778456, 35.04930799450050927 ) ) ;
#29913=ADVANCED_FACE ( 'NONE', ( #13531 ), #23155, .T. ) ;
#29920=DIRECTION ( 'NONE',  ( 0.000000000000000000, 0.000000000000000000, 1.000000000000000000 ) ) ;
#29933=LINE ( 'NONE', #24669, #100 ) ;
#29939=DIRECTION ( 'NONE',  ( 0.000000000000000000, 0.000000000000000000, -1.000000000000000000 ) ) ;
#29948=EDGE_CURVE ( 'NONE', #28978, #1564, #1146, .T. ) ;
#29981=AXIS2_PLACEMENT_3D ( 'NONE', #13225, #22888, #10429 ) ;
#30165=CARTESIAN_POINT ( 'NONE',  ( 21.09785597605719332, 30.56554579224779644, 21.04930799450051282 ) ) ;
#30183=EDGE_CURVE ( 'NONE', #12727, #13855, #29933, .T. ) ;
#30204=PRODUCT_CONTEXT ( 'NONE', #9722, 'mechanical' ) ;
#30262=ORIENTED_EDGE ( 'NONE', *, *, #10158, .T. ) ;
#30345=CARTESIAN_POINT ( 'NONE',  ( 21.09785597605719687, 30.56454579224779522, 14.54930799450051460 ) ) ;
#30358=EDGE_LOOP ( 'NONE', ( #31108, #19193, #20009, #25572 ) ) ;
#30366=VERTEX_POINT ( 'NONE', #3919 ) ;
#30367=DIRECTION ( 'NONE',  ( 0.000000000000000000, -0.000000000000000000, 1.000000000000000000 ) ) ;
#30374=AXIS2_PLACEMENT_3D ( 'NONE', #9272, #24205, #4509 ) ;
#30390=AXIS2_PLACEMENT_3D ( 'NONE', #1226, #24038, #4181 ) ;
#30413=LINE ( 'NONE', #10070, #16108 ) ;
#30430=VECTOR ( 'NONE', #25217, 1000.000000000000000 ) ;
#30432=CIRCLE ( 'NONE', #14194, 2.923537884824412014 ) ;
#30447=VERTEX_POINT ( 'NONE', #14751 ) ;
#30450=AXIS2_PLACEMENT_3D ( 'NONE', #9314, #9647, #19640 ) ;
#30462=ORIENTED_EDGE ( 'NONE', *, *, #29948, .F. ) ;
#30484=EDGE_CURVE ( 'NONE', #12175, #1564, #11800, .T. ) ;
#30501=AXIS2_PLACEMENT_3D ( 'NONE', #23254, #768, #20785 ) ;
#30556=ORIENTED_EDGE ( 'NONE', *, *, #6749, .T. ) ;
#30582=ORIENTED_EDGE ( 'NONE', *, *, #2924, .T. ) ;
#30624=ORIENTED_EDGE ( 'NONE', *, *, #11522, .F. ) ;
#30649=PLANE ( 'NONE',  #10595 ) ;
#30657=ORIENTED_EDGE ( 'NONE', *, *, #23389, .T. ) ;
#30669=ORIENTED_EDGE ( 'NONE', *, *, #22438, .F. ) ;
#30736=EDGE_CURVE ( 'NONE', #19811, #23803, #25731, .T. ) ;
#30791=DIRECTION ( 'NONE',  ( -0.000000000000000000, 1.000000000000000000, -0.000000000000000000 ) ) ;
#30797=DIRECTION ( 'NONE',  ( -1.000000000000000000, 0.000000000000000000, -1.110223024625155594E-14 ) ) ;
#30811=VERTEX_POINT ( 'NONE', #31777 ) ;
#30832=ORIENTED_EDGE ( 'NONE', *, *, #26795, .T. ) ;
#30853=DIRECTION ( 'NONE',  ( 0.000000000000000000, 0.000000000000000000, -1.000000000000000000 ) ) ;
#30879=ORIENTED_EDGE ( 'NONE', *, *, #26696, .F. ) ;
#30924=( LENGTH_UNIT ( ) NAMED_UNIT ( * ) SI_UNIT ( .MILLI., .METRE. ) );
#30930=CARTESIAN_POINT ( 'NONE',  ( -4.902144023942810236, 30.56554579224779644, 47.04930799450042400 ) ) ;
#30969=DIRECTION ( 'NONE',  ( 0.000000000000000000, 1.000000000000000000, 0.000000000000000000 ) ) ;
#30973=CARTESIAN_POINT ( 'NONE',  ( 21.09785597605719687, 25.76454579224776964, 15.54930799450051460 ) ) ;
#30996=VERTEX_POINT ( 'NONE', #7652 ) ;
#31015=CARTESIAN_POINT ( 'NONE',  ( 21.09785597605719332, 40.56454579224780588, 47.04930799450051637 ) ) ;
#31027=EDGE_CURVE ( 'NONE', #3952, #18274, #252, .T. ) ;
#31032=DIRECTION ( 'NONE',  ( 0.000000000000000000, -1.000000000000000000, 0.000000000000000000 ) ) ;
#31080=CARTESIAN_POINT ( 'NONE',  ( 21.09785597605719332, 30.56454579224779522, 79.54930799450052348 ) ) ;
#31107=LINE ( 'NONE', #8612, #26137 ) ;
#31108=ORIENTED_EDGE ( 'NONE', *, *, #1779, .F. ) ;
#31129=FACE_BOUND ( 'NONE', #10768, .T. ) ;
#31131=CARTESIAN_POINT ( 'NONE',  ( 21.09785597605719332, 25.56454579224779877, 58.84930799450049221 ) ) ;
#31144=DIRECTION ( 'NONE',  ( -0.000000000000000000, -1.000000000000000000, -0.000000000000000000 ) ) ;
#31145=EDGE_CURVE ( 'NONE', #8289, #10562, #13065, .T. ) ;
#31246=ORIENTED_EDGE ( 'NONE', *, *, #28888, .F. ) ;
#31286=ORIENTED_EDGE ( 'NONE', *, *, #20572, .T. ) ;
#31344=EDGE_CURVE ( 'NONE', #25267, #2286, #9909, .T. ) ;
#31364=CARTESIAN_POINT ( 'NONE',  ( 21.09785597605719332, 30.56454579224779522, 47.04930799450051637 ) ) ;
#31371=ORIENTED_EDGE ( 'NONE', *, *, #23668, .F. ) ;
#31382=AXIS2_PLACEMENT_3D ( 'NONE', #11189, #28915, #8877 ) ;
#31423=ORIENTED_EDGE ( 'NONE', *, *, #27316, .T. ) ;
#31440=DIRECTION ( 'NONE',  ( 0.000000000000000000, -0.000000000000000000, -1.000000000000000000 ) ) ;
#31469=CARTESIAN_POINT ( 'NONE',  ( 21.09785597605719332, 40.56454579224779877, 47.04930799450051637 ) ) ;
#31472=EDGE_LOOP ( 'NONE', ( #26894, #29165 ) ) ;
#31480=ORIENTED_EDGE ( 'NONE', *, *, #9907, .F. ) ;
#31505=DIRECTION ( 'NONE',  ( 0.000000000000000000, 0.000000000000000000, -1.000000000000000000 ) ) ;
#31526=AXIS2_PLACEMENT_3D ( 'NONE', #8314, #30969, #13089 ) ;
#31527=FACE_OUTER_BOUND ( 'NONE', #3304, .T. ) ;
#31530=DIRECTION ( 'NONE',  ( -0.000000000000000000, -1.000000000000000000, -0.000000000000000000 ) ) ;
#31543=CARTESIAN_POINT ( 'NONE',  ( 21.09785597605719332, 25.56454579224779167, 70.54930799450050927 ) ) ;
#31545=AXIS2_PLACEMENT_3D ( 'NONE', #26187, #28506, #1727 ) ;
#31571=CYLINDRICAL_SURFACE ( 'NONE', #24524, 2.500000000000002220 ) ;
#31574=DIRECTION ( 'NONE',  ( -0.000000000000000000, -1.000000000000000000, -0.000000000000000000 ) ) ;
#31601=CARTESIAN_POINT ( 'NONE',  ( 21.09785597605719332, 28.56454579224779877, 47.04930799450051637 ) ) ;
#31609=LINE ( 'NONE', #30973, #27341 ) ;
#31612=( NAMED_UNIT ( * ) PLANE_ANGLE_UNIT ( ) SI_UNIT ( $, .RADIAN. ) );
#31614=FACE_OUTER_BOUND ( 'NONE', #26984, .T. ) ;
#31633=DIRECTION ( 'NONE',  ( -0.000000000000000000, 1.000000000000000000, -0.000000000000000000 ) ) ;
#31641=CARTESIAN_POINT ( 'NONE',  ( 21.09785597605719332, 43.56454579224774193, 17.04930799450051637 ) ) ;
#31665=FACE_OUTER_BOUND ( 'NONE', #21584, .T. ) ;
#31690=CARTESIAN_POINT ( 'NONE',  ( 21.09785597605719687, 42.30003263981368633, 17.04930799450051637 ) ) ;
#31740=VERTEX_POINT ( 'NONE', #17405 ) ;
#31759=DIRECTION ( 'NONE',  ( 0.000000000000000000, -1.000000000000000000, 0.000000000000000000 ) ) ;
#31777=CARTESIAN_POINT ( 'NONE',  ( 21.09785597605719332, 25.76454579224776964, 15.54930799450051460 ) ) ;
#31799=EDGE_LOOP ( 'NONE', ( #277, #24104, #15875, #11924 ) ) ;
#31812=DIRECTION ( 'NONE',  ( 0.000000000000000000, 1.000000000000000000, 0.000000000000000000 ) ) ;
#31816=CARTESIAN_POINT ( 'NONE',  ( 21.09785597605719332, 25.76454579224781227, 35.04930799450050927 ) ) ;
#31830=ADVANCED_FACE ( 'NONE', ( #22331 ), #25410, .T. ) ;
#31842=DIRECTION ( 'NONE',  ( 0.000000000000000000, 0.000000000000000000, 1.000000000000000000 ) ) ;
#31857=EDGE_LOOP ( 'NONE', ( #31371, #9703, #3352, #686 ) ) ;
#31889=DIRECTION ( 'NONE',  ( 0.000000000000000000, 0.000000000000000000, 1.000000000000000000 ) ) ;
#31927=DIRECTION ( 'NONE',  ( -0.000000000000000000, -1.000000000000000000, -0.000000000000000000 ) ) ;
#31930=LINE ( 'NONE', #2389, #6843 ) ;
#31996=CIRCLE ( 'NONE', #5811, 13.00000000000000533 ) ;
#32006=CARTESIAN_POINT ( 'NONE',  ( 21.09785597605719332, 25.56454579224779167, 18.54930799450051282 ) ) ;
#32046=DIRECTION ( 'NONE',  ( 0.000000000000000000, 0.000000000000000000, 1.000000000000000000 ) ) ;
#32093=ADVANCED_FACE ( 'NONE', ( #7999 ), #28341, .T. ) ;
#32096=CARTESIAN_POINT ( 'NONE',  ( 21.09785597605719332, 28.56454579224779877, 47.04930799450051637 ) ) ;
#32101=EDGE_CURVE ( 'NONE', #10562, #7332, #18093, .T. ) ;
#32123=AXIS2_PLACEMENT_3D ( 'NONE', #17882, #2136, #22145 ) ;
#32160=VERTEX_POINT ( 'NONE', #9565 ) ;
#32168=ORIENTED_EDGE ( 'NONE', *, *, #16380, .T. ) ;
#32170=CARTESIAN_POINT ( 'NONE',  ( 21.09785597605719332, 40.56454579224780588, 47.04930799450051637 ) ) ;
#32202=CIRCLE ( 'NONE', #18044, 16.99999999999999289 ) ;
#32208=DIRECTION ( 'NONE',  ( 0.000000000000000000, -0.000000000000000000, -1.000000000000000000 ) ) ;
#32236=AXIS2_PLACEMENT_3D ( 'NONE', #11409, #5688, #30797 ) ;
#32261=ORIENTED_EDGE ( 'NONE', *, *, #18554, .T. ) ;
#32265=DIRECTION ( 'NONE',  ( 0.000000000000000000, -0.7071067811865383579, -0.7071067811865566766 ) ) ;
#32284=EDGE_LOOP ( 'NONE', ( #5435, #15885, #21085, #8786 ) ) ;
#32288=DIRECTION ( 'NONE',  ( 0.000000000000000000, 0.7071067811865474617, 0.7071067811865474617 ) ) ;
#32324=ORIENTED_EDGE ( 'NONE', *, *, #16298, .F. ) ;
#32351=FACE_OUTER_BOUND ( 'NONE', #25436, .T. ) ;
#32357=EDGE_CURVE ( 'NONE', #23803, #19744, #8145, .T. ) ;
#32361=CARTESIAN_POINT ( 'NONE',  ( 21.09785597605719687, 30.56454579224779522, 78.34930799450049221 ) ) ;
#32392=DIRECTION ( 'NONE',  ( -0.000000000000000000, -1.000000000000000000, -0.000000000000000000 ) ) ;
#32397=EDGE_LOOP ( 'NONE', ( #17702, #29380 ) ) ;
#32413=ORIENTED_EDGE ( 'NONE', *, *, #26413, .F. ) ;
#32425=CARTESIAN_POINT ( 'NONE',  ( 47.09785597605719687, 30.56454579224779522, 49.54930799450078638 ) ) ;
#32445=CIRCLE ( 'NONE', #31382, 2.923537884824412014 ) ;
#32451=DIRECTION ( 'NONE',  ( 0.000000000000000000, -0.1908089953765421121, -0.9816271834476645308 ) ) ;
#32463=CARTESIAN_POINT ( 'NONE',  ( 21.09785597605719332, 30.56454579224779522, 47.04930799450051637 ) ) ;
#32481=CIRCLE ( 'NONE', #30374, 19.18998195308981636 ) ;
#32485=AXIS2_PLACEMENT_3D ( 'NONE', #17072, #4603, #27089 ) ;
#32496=ORIENTED_EDGE ( 'NONE', *, *, #22252, .F. ) ;
#32516=COLOUR_RGB('Light Blue',0.38,0.62,0.78);
#32517=FILL_AREA_STYLE_COLOUR('',#32516);
#32518=FILL_AREA_STYLE('',(#32517));
#32519=SURFACE_STYLE_FILL_AREA(#32518);
#32520=SURFACE_SIDE_STYLE('',(#32519));
#32521=SURFACE_STYLE_USAGE(.BOTH.,#32520);
#32522=PRESENTATION_STYLE_ASSIGNMENT((#32521));
ENDSEC;
END-ISO-10303-21;
